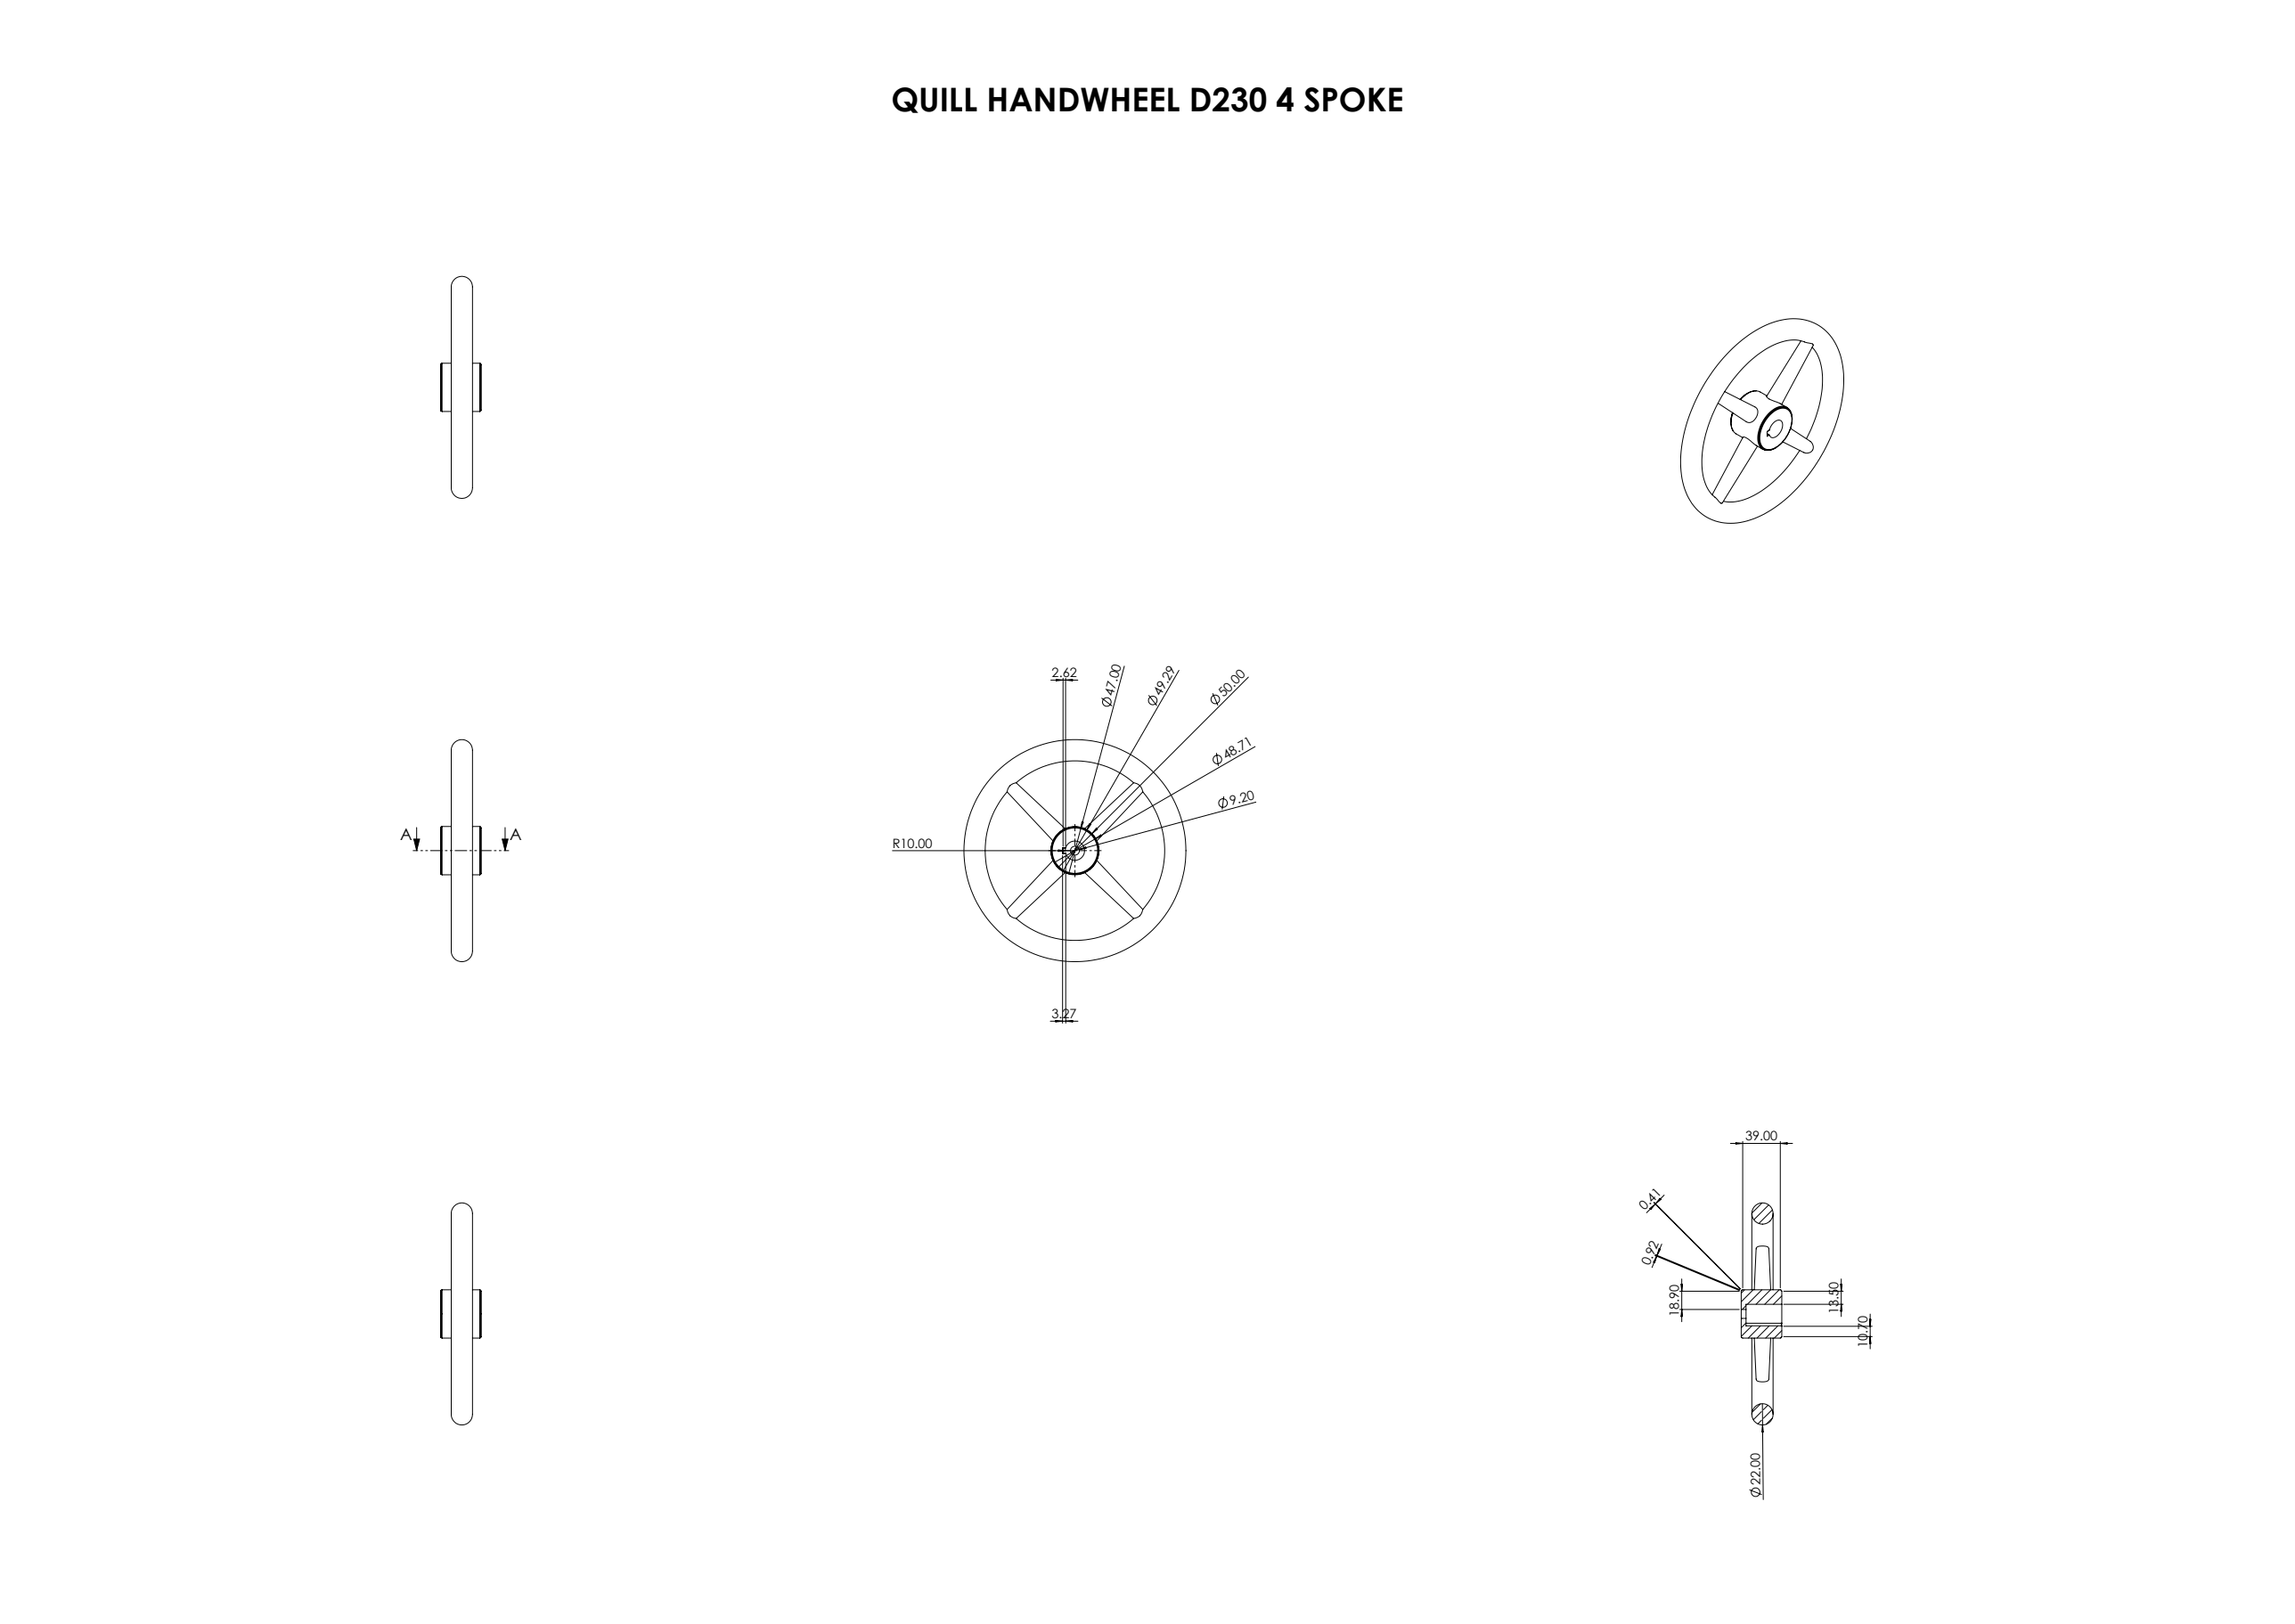
ISO-10303-21;
HEADER;
/* Generated by software containing ST-Developer
 * from STEP Tools, Inc. (www.steptools.com) 
 */

FILE_DESCRIPTION(
/* description */ (''),
/* implementation_level */ '2;1');

FILE_NAME(
/* name */ '09_Quill_Handwheel_D230_4_Spoke.step',
/* time_stamp */ '2026-10-26T03:50:32-07:00',
/* author */ (''),
/* organization */ (''),
/* preprocessor_version */ 'ST-DEVELOPER v20.2',
/* originating_system */ 'Autodesk Translation Framework v15.15.0.0',
/* authorisation */ '');

FILE_SCHEMA (('AUTOMOTIVE_DESIGN { 1 0 10303 214 3 1 1 }'));
ENDSEC;

DATA;
#10=MECHANICAL_DESIGN_GEOMETRIC_PRESENTATION_REPRESENTATION('',(#1046),#76660);
#421=B_SPLINE_CURVE_WITH_KNOTS('',3,(#49844,#49845,#49846,#49847,#49848,
#49849,#49850,#49851,#49852,#49853,#49854,#49855,#49856,#49857,#49858,#49859,
#49860,#49861),.UNSPECIFIED.,.F.,.F.,(4,2,2,2,2,2,2,2,4),(0.,0.33755490943604,
0.675109818872081,1.01195490866249,1.34879999845289,1.6856450882433,2.02249017803371,
2.36004508746975,2.69759999690579),.UNSPECIFIED.);
#422=B_SPLINE_CURVE_WITH_KNOTS('',3,(#49862,#49863,#49864,#49865,#49866,
#49867,#49868,#49869,#49870,#49871,#49872,#49873,#49874,#49875,#49876,#49877,
#49878,#49879),.UNSPECIFIED.,.F.,.F.,(4,2,2,2,2,2,2,2,4),(2.69759999690579,
3.03515490634183,3.37270981577787,3.70955490556828,4.04639999535868,4.38324508514909,
4.72009017493949,5.05764508437554,5.39519999381158),.UNSPECIFIED.);
#423=B_SPLINE_CURVE_WITH_KNOTS('',3,(#49882,#49883,#49884,#49885,#49886,
#49887,#49888,#49889,#49890,#49891,#49892,#49893,#49894,#49895,#49896,#49897,
#49898,#49899),.UNSPECIFIED.,.F.,.F.,(4,2,2,2,2,2,2,2,4),(0.,0.337554909436041,
0.675109818872083,1.01195490866249,1.34879999845289,1.6856450882433,2.0224901780337,
2.36004508746974,2.69759999690578),.UNSPECIFIED.);
#424=B_SPLINE_CURVE_WITH_KNOTS('',3,(#49900,#49901,#49902,#49903,#49904,
#49905,#49906,#49907,#49908,#49909,#49910,#49911,#49912,#49913,#49914,#49915,
#49916,#49917),.UNSPECIFIED.,.F.,.F.,(4,2,2,2,2,2,2,2,4),(2.69759999690578,
3.03515490634183,3.37270981577787,3.70955490556827,4.04639999535868,4.38324508514908,
4.72009017493949,5.05764508437553,5.39519999381157),.UNSPECIFIED.);
#425=B_SPLINE_CURVE_WITH_KNOTS('',3,(#49920,#49921,#49922,#49923,#49924,
#49925,#49926,#49927,#49928,#49929,#49930,#49931,#49932,#49933,#49934,#49935,
#49936,#49937),.UNSPECIFIED.,.F.,.F.,(4,2,2,2,2,2,2,2,4),(0.,0.337554909436041,
0.675109818872081,1.01195490866249,1.3487999984529,1.6856450882433,2.02249017803371,
2.36004508746975,2.69759999690579),.UNSPECIFIED.);
#426=B_SPLINE_CURVE_WITH_KNOTS('',3,(#49938,#49939,#49940,#49941,#49942,
#49943,#49944,#49945,#49946,#49947,#49948,#49949,#49950,#49951,#49952,#49953,
#49954,#49955),.UNSPECIFIED.,.F.,.F.,(4,2,2,2,2,2,2,2,4),(2.69759999690579,
3.03515490634183,3.37270981577787,3.70955490556828,4.04639999535869,4.3832450851491,
4.7200901749395,5.05764508437554,5.39519999381158),.UNSPECIFIED.);
#427=B_SPLINE_CURVE_WITH_KNOTS('',3,(#49958,#49959,#49960,#49961,#49962,
#49963,#49964,#49965,#49966,#49967,#49968,#49969,#49970,#49971,#49972,#49973,
#49974,#49975),.UNSPECIFIED.,.F.,.F.,(4,2,2,2,2,2,2,2,4),(0.,0.337554909436041,
0.675109818872081,1.01195490866249,1.3487999984529,1.6856450882433,2.02249017803371,
2.36004508746975,2.69759999690579),.UNSPECIFIED.);
#428=B_SPLINE_CURVE_WITH_KNOTS('',3,(#49976,#49977,#49978,#49979,#49980,
#49981,#49982,#49983,#49984,#49985,#49986,#49987,#49988,#49989,#49990,#49991,
#49992,#49993),.UNSPECIFIED.,.F.,.F.,(4,2,2,2,2,2,2,2,4),(2.69759999690579,
3.03515490634183,3.37270981577787,3.70955490556828,4.04639999535869,4.3832450851491,
4.72009017493951,5.05764508437555,5.39519999381159),.UNSPECIFIED.);
#429=B_SPLINE_CURVE_WITH_KNOTS('',3,(#50065,#50066,#50067,#50068,#50069,
#50070,#50071,#50072,#50073,#50074,#50075,#50076,#50077,#50078,#50079,#50080),
 .UNSPECIFIED.,.F.,.F.,(4,2,2,2,2,2,2,4),(-4.30443928379571,-4.2860545404295,
-4.18302089376354,-4.02031324727212,-3.73577474040229,-3.47881030687683,
-3.26117067957846,-3.22870524423984),.UNSPECIFIED.);
#430=B_SPLINE_CURVE_WITH_KNOTS('',3,(#50082,#50083,#50084,#50085,#50086,
#50087,#50088,#50089,#50090,#50091,#50092,#50093,#50094,#50095),
 .UNSPECIFIED.,.F.,.F.,(4,2,2,2,2,2,4),(-1.07597467085911,-1.02250399542755,
-0.791813858983204,-0.526066025069406,-0.242334063735881,-0.0987908890199728,
0.),.UNSPECIFIED.);
#431=B_SPLINE_CURVE_WITH_KNOTS('',3,(#50096,#50097,#50098,#50099,#50100,
#50101,#50102,#50103,#50104,#50105,#50106,#50107,#50108,#50109,#50110,#50111,
#50112,#50113,#50114,#50115,#50116,#50117,#50118,#50119),.UNSPECIFIED.,
 .F.,.F.,(4,2,2,2,2,2,2,2,2,2,2,4),(-3.22870524423984,-3.04034029687005,
-2.77983245466332,-2.48572420120637,-2.29812682077172,-2.18914179422406,
-2.09440056074871,-1.97639597697234,-1.7640763751916,-1.47308567187965,
-1.23740056701131,-1.07597467085911),.UNSPECIFIED.);
#432=B_SPLINE_CURVE_WITH_KNOTS('',3,(#50124,#50125,#50126,#50127,#50128,
#50129,#50130,#50131,#50132,#50133,#50134,#50135,#50136,#50137,#50138,#50139),
 .UNSPECIFIED.,.F.,.F.,(4,2,2,2,2,2,2,4),(-4.30443928376566,-4.28605454039955,
-4.18302089373508,-4.02031324724582,-3.73577474037948,-3.47881030685707,
-3.2611706795612,-3.22870524422297),.UNSPECIFIED.);
#433=B_SPLINE_CURVE_WITH_KNOTS('',3,(#50141,#50142,#50143,#50144,#50145,
#50146,#50147,#50148,#50149,#50150,#50151,#50152,#50153,#50154),
 .UNSPECIFIED.,.F.,.F.,(4,2,2,2,2,2,4),(-1.07597467085728,-1.02250399542586,
-0.791813858982145,-0.526066025068897,-0.242334063735757,-0.0987908890199458,
0.),.UNSPECIFIED.);
#434=B_SPLINE_CURVE_WITH_KNOTS('',3,(#50155,#50156,#50157,#50158,#50159,
#50160,#50161,#50162,#50163,#50164,#50165,#50166,#50167,#50168,#50169,#50170,
#50171,#50172,#50173,#50174,#50175,#50176,#50177,#50178),.UNSPECIFIED.,
 .F.,.F.,(4,2,2,2,2,2,2,2,2,2,2,4),(-3.22870524422297,-3.0403402968552,
-2.7798324546511,-2.48572420119689,-2.29812682076393,-2.18914179421705,
-2.09440056074233,-1.97639597696673,-1.76407637518704,-1.47308567187632,
-1.23740056700891,-1.07597467085728),.UNSPECIFIED.);
#435=B_SPLINE_CURVE_WITH_KNOTS('',3,(#50183,#50184,#50185,#50186,#50187,
#50188,#50189,#50190,#50191,#50192,#50193,#50194,#50195,#50196,#50197,#50198),
 .UNSPECIFIED.,.F.,.F.,(4,2,2,2,2,2,2,4),(-4.30443928371459,-4.28605454034862,
-4.18302089368667,-4.02031324720125,-3.73577474034113,-3.47881030682397,
-3.2611706795323,-3.22870524419465),.UNSPECIFIED.);
#436=B_SPLINE_CURVE_WITH_KNOTS('',3,(#50200,#50201,#50202,#50203,#50204,
#50205,#50206,#50207,#50208,#50209,#50210,#50211,#50212,#50213),
 .UNSPECIFIED.,.F.,.F.,(4,2,2,2,2,2,4),(-1.07597467085434,-1.02250399542317,
-0.791813858980425,-0.526066025068098,-0.242334063735552,-0.098790889019902,
0.),.UNSPECIFIED.);
#437=B_SPLINE_CURVE_WITH_KNOTS('',3,(#50214,#50215,#50216,#50217,#50218,
#50219,#50220,#50221,#50222,#50223,#50224,#50225,#50226,#50227,#50228,#50229,
#50230,#50231,#50232,#50233,#50234,#50235,#50236,#50237),.UNSPECIFIED.,
 .F.,.F.,(4,2,2,2,2,2,2,2,2,2,2,4),(-3.22870524419465,-3.04034029683025,
-2.77983245463047,-2.48572420118091,-2.2981268207507,-2.18914179420531,
-2.09440056073169,-1.97639597695723,-1.76407637517944,-1.47308567187093,
-1.23740056700507,-1.07597467085434),.UNSPECIFIED.);
#438=B_SPLINE_CURVE_WITH_KNOTS('',3,(#50242,#50243,#50244,#50245,#50246,
#50247,#50248,#50249,#50250,#50251,#50252,#50253,#50254,#50255,#50256,#50257),
 .UNSPECIFIED.,.F.,.F.,(4,2,2,2,2,2,2,4),(-4.30443928358367,-4.28605454021807,
-4.18302089356202,-4.02031324708534,-3.73577474023997,-3.47881030673541,
-3.26117067945383,-3.22870524411765),.UNSPECIFIED.);
#439=B_SPLINE_CURVE_WITH_KNOTS('',3,(#50259,#50260,#50261,#50262,#50263,
#50264,#50265,#50266,#50267,#50268,#50269,#50270,#50271,#50272),
 .UNSPECIFIED.,.F.,.F.,(4,2,2,2,2,2,4),(-1.07597467084362,-1.02250399541335,
-0.791813858973979,-0.526066025064686,-0.242334063734663,-0.0987908890197505,
0.),.UNSPECIFIED.);
#440=B_SPLINE_CURVE_WITH_KNOTS('',3,(#50273,#50274,#50275,#50276,#50277,
#50278,#50279,#50280,#50281,#50282,#50283,#50284,#50285,#50286,#50287,#50288,
#50289,#50290,#50291,#50292,#50293,#50294,#50295,#50296),.UNSPECIFIED.,
 .F.,.F.,(4,2,2,2,2,2,2,2,2,2,2,4),(-3.22870524411765,-3.04034029676145,
-2.77983245457245,-2.48572420113423,-2.29812682071072,-2.18914179416892,
-2.0944005606982,-1.976395976927,-1.76407637515459,-1.47308567185275,-1.23740056699153,
-1.07597467084362),.UNSPECIFIED.);
#1006=SHAPE_REPRESENTATION_RELATIONSHIP('SRR','None',#76743,#1026);
#1026=ADVANCED_BREP_SHAPE_REPRESENTATION('',(#1066),#76647);
#1046=STYLED_ITEM('',(#76899),#1066);
#1066=MANIFOLD_SOLID_BREP('Handwheel',#26671);
#1085=TOROIDAL_SURFACE('',#27865,10.4,1.1);
#1099=ELLIPSE('',#27852,1.41421356237309,1.);
#1100=ELLIPSE('',#27854,1.41421356237308,1.);
#1265=CYLINDRICAL_SURFACE('',#27831,2.5);
#1266=CYLINDRICAL_SURFACE('',#27859,1.);
#1267=CYLINDRICAL_SURFACE('',#27872,0.46);
#1628=FACE_BOUND('',#4742,.T.);
#1629=FACE_BOUND('',#4743,.T.);
#1630=FACE_BOUND('',#4744,.T.);
#1631=FACE_BOUND('',#4745,.T.);
#1632=FACE_BOUND('',#4751,.T.);
#1633=FACE_BOUND('',#4754,.T.);
#1634=FACE_BOUND('',#4769,.T.);
#1935=PLANE('',#27845);
#1936=PLANE('',#27849);
#1937=PLANE('',#27851);
#1938=PLANE('',#27853);
#1939=PLANE('',#27855);
#1940=PLANE('',#27856);
#1941=PLANE('',#27857);
#1942=PLANE('',#27858);
#1943=PLANE('',#27874);
#3113=FACE_OUTER_BOUND('',#4740,.T.);
#3114=FACE_OUTER_BOUND('',#4741,.T.);
#3115=FACE_OUTER_BOUND('',#4746,.T.);
#3116=FACE_OUTER_BOUND('',#4747,.T.);
#3117=FACE_OUTER_BOUND('',#4748,.T.);
#3118=FACE_OUTER_BOUND('',#4749,.T.);
#3119=FACE_OUTER_BOUND('',#4750,.T.);
#3120=FACE_OUTER_BOUND('',#4752,.T.);
#3121=FACE_OUTER_BOUND('',#4753,.T.);
#3122=FACE_OUTER_BOUND('',#4755,.T.);
#3123=FACE_OUTER_BOUND('',#4756,.T.);
#3124=FACE_OUTER_BOUND('',#4757,.T.);
#3125=FACE_OUTER_BOUND('',#4758,.T.);
#3126=FACE_OUTER_BOUND('',#4759,.T.);
#3127=FACE_OUTER_BOUND('',#4760,.T.);
#3128=FACE_OUTER_BOUND('',#4761,.T.);
#3129=FACE_OUTER_BOUND('',#4762,.T.);
#3130=FACE_OUTER_BOUND('',#4763,.T.);
#3131=FACE_OUTER_BOUND('',#4764,.T.);
#3132=FACE_OUTER_BOUND('',#4765,.T.);
#3133=FACE_OUTER_BOUND('',#4766,.T.);
#3134=FACE_OUTER_BOUND('',#4767,.T.);
#3135=FACE_OUTER_BOUND('',#4768,.T.);
#4740=EDGE_LOOP('',(#20043,#20044,#20045,#20046,#20047,#20048));
#4741=EDGE_LOOP('',(#20049,#20050,#20051,#20052,#20053,#20054));
#4742=EDGE_LOOP('',(#20055,#20056));
#4743=EDGE_LOOP('',(#20057,#20058));
#4744=EDGE_LOOP('',(#20059,#20060));
#4745=EDGE_LOOP('',(#20061,#20062));
#4746=EDGE_LOOP('',(#20063,#20064,#20065,#20066,#20067,#20068));
#4747=EDGE_LOOP('',(#20069,#20070,#20071,#20072,#20073,#20074));
#4748=EDGE_LOOP('',(#20075,#20076,#20077,#20078,#20079,#20080));
#4749=EDGE_LOOP('',(#20081,#20082,#20083,#20084,#20085));
#4750=EDGE_LOOP('',(#20086));
#4751=EDGE_LOOP('',(#20087));
#4752=EDGE_LOOP('',(#20088,#20089,#20090,#20091,#20092));
#4753=EDGE_LOOP('',(#20093));
#4754=EDGE_LOOP('',(#20094,#20095,#20096,#20097));
#4755=EDGE_LOOP('',(#20098,#20099,#20100,#20101));
#4756=EDGE_LOOP('',(#20102,#20103,#20104,#20105));
#4757=EDGE_LOOP('',(#20106,#20107,#20108,#20109));
#4758=EDGE_LOOP('',(#20110,#20111,#20112,#20113));
#4759=EDGE_LOOP('',(#20114,#20115,#20116,#20117));
#4760=EDGE_LOOP('',(#20118,#20119,#20120,#20121));
#4761=EDGE_LOOP('',(#20122,#20123,#20124,#20125,#20126,#20127));
#4762=EDGE_LOOP('',(#20128,#20129,#20130,#20131,#20132,#20133,#20134));
#4763=EDGE_LOOP('',(#20135,#20136,#20137,#20138,#20139,#20140,#20141));
#4764=EDGE_LOOP('',(#20142,#20143,#20144,#20145,#20146,#20147,#20148));
#4765=EDGE_LOOP('',(#20149,#20150,#20151,#20152,#20153,#20154,#20155));
#4766=EDGE_LOOP('',(#20156,#20157,#20158,#20159,#20160,#20161,#20162,#20163,
#20164,#20165,#20166,#20167,#20168,#20169,#20170,#20171,#20172,#20173,#20174,
#20175,#20176,#20177,#20178,#20179));
#4767=EDGE_LOOP('',(#20180,#20181,#20182,#20183));
#4768=EDGE_LOOP('',(#20184,#20185,#20186,#20187));
#4769=EDGE_LOOP('',(#20188));
#6066=CIRCLE('',#27827,2.46464466094067);
#6067=CIRCLE('',#27828,2.46464466094067);
#6068=CIRCLE('',#27829,2.5);
#6069=CIRCLE('',#27830,2.5);
#6070=CIRCLE('',#27832,2.5);
#6071=CIRCLE('',#27833,2.5);
#6072=CIRCLE('',#27835,2.43535533905933);
#6073=CIRCLE('',#27836,2.43535533905933);
#6074=CIRCLE('',#27838,2.46464466094067);
#6075=CIRCLE('',#27839,2.46464466094067);
#6076=CIRCLE('',#27841,2.43535533905933);
#6077=CIRCLE('',#27842,2.43535533905933);
#6078=CIRCLE('',#27844,2.35);
#6079=CIRCLE('',#27846,0.46);
#6080=CIRCLE('',#27848,2.35);
#6081=CIRCLE('',#27850,1.);
#6082=CIRCLE('',#27860,1.);
#6083=CIRCLE('',#27866,1.1);
#6084=CIRCLE('',#27867,9.3);
#6085=CIRCLE('',#27868,9.3);
#6086=CIRCLE('',#27869,9.3);
#6087=CIRCLE('',#27870,9.3);
#6088=CIRCLE('',#27871,9.3);
#6089=CIRCLE('',#27873,0.46);
#7429=LINE('',#49832,#9585);
#7430=LINE('',#49838,#9586);
#7431=LINE('',#49999,#9587);
#7432=LINE('',#50002,#9588);
#7433=LINE('',#50008,#9589);
#7434=LINE('',#50014,#9590);
#7435=LINE('',#50022,#9591);
#7436=LINE('',#50026,#9592);
#7437=LINE('',#50030,#9593);
#7438=LINE('',#50031,#9594);
#7439=LINE('',#50035,#9595);
#7440=LINE('',#50037,#9596);
#7441=LINE('',#50042,#9597);
#7442=LINE('',#50043,#9598);
#7443=LINE('',#50045,#9599);
#7444=LINE('',#50048,#9600);
#7445=LINE('',#50050,#9601);
#7446=LINE('',#50051,#9602);
#7447=LINE('',#50054,#9603);
#7448=LINE('',#50055,#9604);
#7449=LINE('',#50058,#9605);
#7450=LINE('',#50059,#9606);
#7451=LINE('',#50120,#9607);
#7452=LINE('',#50179,#9608);
#7453=LINE('',#50238,#9609);
#7454=LINE('',#50297,#9610);
#7455=LINE('',#50309,#9611);
#9585=VECTOR('',#32030,2.48232233047034);
#9586=VECTOR('',#32037,2.5);
#9587=VECTOR('',#32048,2.45);
#9588=VECTOR('',#32051,2.48232233047034);
#9589=VECTOR('',#32058,2.45);
#9590=VECTOR('',#32065,2.39267766952966);
#9591=VECTOR('',#32076,2.39267766952966);
#9592=VECTOR('',#32079,1.);
#9593=VECTOR('',#32082,1.);
#9594=VECTOR('',#32083,1.);
#9595=VECTOR('',#32086,1.);
#9596=VECTOR('',#32089,1.);
#9597=VECTOR('',#32094,1.);
#9598=VECTOR('',#32095,1.);
#9599=VECTOR('',#32098,1.);
#9600=VECTOR('',#32101,1.);
#9601=VECTOR('',#32102,1.);
#9602=VECTOR('',#32103,1.);
#9603=VECTOR('',#32106,1.);
#9604=VECTOR('',#32107,1.);
#9605=VECTOR('',#32110,1.);
#9606=VECTOR('',#32111,1.);
#9607=VECTOR('',#32118,0.775);
#9608=VECTOR('',#32121,0.775);
#9609=VECTOR('',#32124,0.775000000000002);
#9610=VECTOR('',#32127,0.774999999999997);
#9611=VECTOR('',#32146,0.46);
#11797=VERTEX_POINT('',#49827);
#11798=VERTEX_POINT('',#49828);
#11799=VERTEX_POINT('',#49831);
#11800=VERTEX_POINT('',#49833);
#11801=VERTEX_POINT('',#49837);
#11802=VERTEX_POINT('',#49839);
#11803=VERTEX_POINT('',#49842);
#11804=VERTEX_POINT('',#49843);
#11805=VERTEX_POINT('',#49880);
#11806=VERTEX_POINT('',#49881);
#11807=VERTEX_POINT('',#49918);
#11808=VERTEX_POINT('',#49919);
#11809=VERTEX_POINT('',#49956);
#11810=VERTEX_POINT('',#49957);
#11811=VERTEX_POINT('',#49995);
#11812=VERTEX_POINT('',#49996);
#11813=VERTEX_POINT('',#50001);
#11814=VERTEX_POINT('',#50003);
#11815=VERTEX_POINT('',#50007);
#11816=VERTEX_POINT('',#50009);
#11817=VERTEX_POINT('',#50013);
#11818=VERTEX_POINT('',#50017);
#11819=VERTEX_POINT('',#50020);
#11820=VERTEX_POINT('',#50024);
#11821=VERTEX_POINT('',#50025);
#11822=VERTEX_POINT('',#50027);
#11823=VERTEX_POINT('',#50029);
#11824=VERTEX_POINT('',#50033);
#11825=VERTEX_POINT('',#50034);
#11826=VERTEX_POINT('',#50039);
#11827=VERTEX_POINT('',#50041);
#11828=VERTEX_POINT('',#50047);
#11829=VERTEX_POINT('',#50049);
#11830=VERTEX_POINT('',#50053);
#11831=VERTEX_POINT('',#50057);
#11832=VERTEX_POINT('',#50063);
#11833=VERTEX_POINT('',#50064);
#11834=VERTEX_POINT('',#50081);
#11835=VERTEX_POINT('',#50122);
#11836=VERTEX_POINT('',#50123);
#11837=VERTEX_POINT('',#50140);
#11838=VERTEX_POINT('',#50181);
#11839=VERTEX_POINT('',#50182);
#11840=VERTEX_POINT('',#50199);
#11841=VERTEX_POINT('',#50240);
#11842=VERTEX_POINT('',#50241);
#11843=VERTEX_POINT('',#50258);
#11844=VERTEX_POINT('',#50299);
#11845=VERTEX_POINT('',#50307);
#14744=EDGE_CURVE('',#11797,#11798,#6066,.T.);
#14745=EDGE_CURVE('',#11798,#11797,#6067,.T.);
#14746=EDGE_CURVE('',#11797,#11799,#7429,.T.);
#14747=EDGE_CURVE('',#11799,#11800,#6068,.T.);
#14748=EDGE_CURVE('',#11800,#11799,#6069,.T.);
#14749=EDGE_CURVE('',#11800,#11801,#7430,.T.);
#14750=EDGE_CURVE('',#11802,#11801,#6070,.T.);
#14751=EDGE_CURVE('',#11801,#11802,#6071,.T.);
#14752=EDGE_CURVE('',#11803,#11804,#421,.T.);
#14753=EDGE_CURVE('',#11804,#11803,#422,.T.);
#14754=EDGE_CURVE('',#11805,#11806,#423,.T.);
#14755=EDGE_CURVE('',#11806,#11805,#424,.T.);
#14756=EDGE_CURVE('',#11807,#11808,#425,.T.);
#14757=EDGE_CURVE('',#11808,#11807,#426,.T.);
#14758=EDGE_CURVE('',#11809,#11810,#427,.T.);
#14759=EDGE_CURVE('',#11810,#11809,#428,.T.);
#14760=EDGE_CURVE('',#11811,#11812,#6072,.T.);
#14761=EDGE_CURVE('',#11812,#11811,#6073,.T.);
#14762=EDGE_CURVE('',#11812,#11798,#7431,.T.);
#14763=EDGE_CURVE('',#11802,#11813,#7432,.T.);
#14764=EDGE_CURVE('',#11813,#11814,#6074,.T.);
#14765=EDGE_CURVE('',#11814,#11813,#6075,.T.);
#14766=EDGE_CURVE('',#11814,#11815,#7433,.T.);
#14767=EDGE_CURVE('',#11816,#11815,#6076,.T.);
#14768=EDGE_CURVE('',#11815,#11816,#6077,.T.);
#14769=EDGE_CURVE('',#11816,#11817,#7434,.T.);
#14770=EDGE_CURVE('',#11817,#11817,#6078,.T.);
#14771=EDGE_CURVE('',#11818,#11818,#6079,.T.);
#14772=EDGE_CURVE('',#11819,#11819,#6080,.T.);
#14773=EDGE_CURVE('',#11819,#11811,#7435,.T.);
#14774=EDGE_CURVE('',#11820,#11821,#7436,.T.);
#14775=EDGE_CURVE('',#11822,#11820,#6081,.T.);
#14776=EDGE_CURVE('',#11823,#11822,#7437,.T.);
#14777=EDGE_CURVE('',#11821,#11823,#7438,.T.);
#14778=EDGE_CURVE('',#11824,#11825,#7439,.T.);
#14779=EDGE_CURVE('',#11825,#11820,#1099,.T.);
#14780=EDGE_CURVE('',#11821,#11824,#7440,.T.);
#14781=EDGE_CURVE('',#11822,#11826,#1100,.T.);
#14782=EDGE_CURVE('',#11826,#11827,#7441,.T.);
#14783=EDGE_CURVE('',#11827,#11823,#7442,.T.);
#14784=EDGE_CURVE('',#11827,#11824,#7443,.T.);
#14785=EDGE_CURVE('',#11828,#11827,#7444,.T.);
#14786=EDGE_CURVE('',#11829,#11828,#7445,.T.);
#14787=EDGE_CURVE('',#11824,#11829,#7446,.T.);
#14788=EDGE_CURVE('',#11830,#11826,#7447,.T.);
#14789=EDGE_CURVE('',#11828,#11830,#7448,.T.);
#14790=EDGE_CURVE('',#11829,#11831,#7449,.T.);
#14791=EDGE_CURVE('',#11825,#11831,#7450,.T.);
#14792=EDGE_CURVE('',#11830,#11831,#6082,.T.);
#14793=EDGE_CURVE('',#11832,#11833,#429,.T.);
#14794=EDGE_CURVE('',#11834,#11832,#430,.T.);
#14795=EDGE_CURVE('',#11833,#11834,#431,.T.);
#14796=EDGE_CURVE('',#11833,#11804,#7451,.T.);
#14797=EDGE_CURVE('',#11835,#11836,#432,.T.);
#14798=EDGE_CURVE('',#11837,#11835,#433,.T.);
#14799=EDGE_CURVE('',#11836,#11837,#434,.T.);
#14800=EDGE_CURVE('',#11836,#11806,#7452,.T.);
#14801=EDGE_CURVE('',#11838,#11839,#435,.T.);
#14802=EDGE_CURVE('',#11840,#11838,#436,.T.);
#14803=EDGE_CURVE('',#11839,#11840,#437,.T.);
#14804=EDGE_CURVE('',#11839,#11808,#7453,.T.);
#14805=EDGE_CURVE('',#11841,#11842,#438,.T.);
#14806=EDGE_CURVE('',#11843,#11841,#439,.T.);
#14807=EDGE_CURVE('',#11842,#11843,#440,.T.);
#14808=EDGE_CURVE('',#11842,#11810,#7454,.T.);
#14809=EDGE_CURVE('',#11844,#11844,#6083,.T.);
#14810=EDGE_CURVE('',#11839,#11844,#6084,.T.);
#14811=EDGE_CURVE('',#11836,#11840,#6085,.T.);
#14812=EDGE_CURVE('',#11833,#11837,#6086,.T.);
#14813=EDGE_CURVE('',#11842,#11834,#6087,.T.);
#14814=EDGE_CURVE('',#11844,#11843,#6088,.T.);
#14815=EDGE_CURVE('',#11845,#11845,#6089,.T.);
#14816=EDGE_CURVE('',#11845,#11818,#7455,.T.);
#20043=ORIENTED_EDGE('',*,*,#14744,.T.);
#20044=ORIENTED_EDGE('',*,*,#14745,.T.);
#20045=ORIENTED_EDGE('',*,*,#14746,.T.);
#20046=ORIENTED_EDGE('',*,*,#14747,.T.);
#20047=ORIENTED_EDGE('',*,*,#14748,.T.);
#20048=ORIENTED_EDGE('',*,*,#14746,.F.);
#20049=ORIENTED_EDGE('',*,*,#14747,.F.);
#20050=ORIENTED_EDGE('',*,*,#14748,.F.);
#20051=ORIENTED_EDGE('',*,*,#14749,.T.);
#20052=ORIENTED_EDGE('',*,*,#14750,.F.);
#20053=ORIENTED_EDGE('',*,*,#14751,.F.);
#20054=ORIENTED_EDGE('',*,*,#14749,.F.);
#20055=ORIENTED_EDGE('',*,*,#14752,.T.);
#20056=ORIENTED_EDGE('',*,*,#14753,.T.);
#20057=ORIENTED_EDGE('',*,*,#14754,.T.);
#20058=ORIENTED_EDGE('',*,*,#14755,.T.);
#20059=ORIENTED_EDGE('',*,*,#14756,.T.);
#20060=ORIENTED_EDGE('',*,*,#14757,.T.);
#20061=ORIENTED_EDGE('',*,*,#14758,.T.);
#20062=ORIENTED_EDGE('',*,*,#14759,.T.);
#20063=ORIENTED_EDGE('',*,*,#14760,.F.);
#20064=ORIENTED_EDGE('',*,*,#14761,.F.);
#20065=ORIENTED_EDGE('',*,*,#14762,.T.);
#20066=ORIENTED_EDGE('',*,*,#14744,.F.);
#20067=ORIENTED_EDGE('',*,*,#14745,.F.);
#20068=ORIENTED_EDGE('',*,*,#14762,.F.);
#20069=ORIENTED_EDGE('',*,*,#14750,.T.);
#20070=ORIENTED_EDGE('',*,*,#14751,.T.);
#20071=ORIENTED_EDGE('',*,*,#14763,.T.);
#20072=ORIENTED_EDGE('',*,*,#14764,.T.);
#20073=ORIENTED_EDGE('',*,*,#14765,.T.);
#20074=ORIENTED_EDGE('',*,*,#14763,.F.);
#20075=ORIENTED_EDGE('',*,*,#14764,.F.);
#20076=ORIENTED_EDGE('',*,*,#14765,.F.);
#20077=ORIENTED_EDGE('',*,*,#14766,.T.);
#20078=ORIENTED_EDGE('',*,*,#14767,.F.);
#20079=ORIENTED_EDGE('',*,*,#14768,.F.);
#20080=ORIENTED_EDGE('',*,*,#14766,.F.);
#20081=ORIENTED_EDGE('',*,*,#14767,.T.);
#20082=ORIENTED_EDGE('',*,*,#14768,.T.);
#20083=ORIENTED_EDGE('',*,*,#14769,.T.);
#20084=ORIENTED_EDGE('',*,*,#14770,.T.);
#20085=ORIENTED_EDGE('',*,*,#14769,.F.);
#20086=ORIENTED_EDGE('',*,*,#14770,.F.);
#20087=ORIENTED_EDGE('',*,*,#14771,.T.);
#20088=ORIENTED_EDGE('',*,*,#14772,.T.);
#20089=ORIENTED_EDGE('',*,*,#14773,.T.);
#20090=ORIENTED_EDGE('',*,*,#14760,.T.);
#20091=ORIENTED_EDGE('',*,*,#14761,.T.);
#20092=ORIENTED_EDGE('',*,*,#14773,.F.);
#20093=ORIENTED_EDGE('',*,*,#14772,.F.);
#20094=ORIENTED_EDGE('',*,*,#14774,.F.);
#20095=ORIENTED_EDGE('',*,*,#14775,.F.);
#20096=ORIENTED_EDGE('',*,*,#14776,.F.);
#20097=ORIENTED_EDGE('',*,*,#14777,.F.);
#20098=ORIENTED_EDGE('',*,*,#14778,.T.);
#20099=ORIENTED_EDGE('',*,*,#14779,.T.);
#20100=ORIENTED_EDGE('',*,*,#14774,.T.);
#20101=ORIENTED_EDGE('',*,*,#14780,.T.);
#20102=ORIENTED_EDGE('',*,*,#14776,.T.);
#20103=ORIENTED_EDGE('',*,*,#14781,.T.);
#20104=ORIENTED_EDGE('',*,*,#14782,.T.);
#20105=ORIENTED_EDGE('',*,*,#14783,.T.);
#20106=ORIENTED_EDGE('',*,*,#14777,.T.);
#20107=ORIENTED_EDGE('',*,*,#14783,.F.);
#20108=ORIENTED_EDGE('',*,*,#14784,.T.);
#20109=ORIENTED_EDGE('',*,*,#14780,.F.);
#20110=ORIENTED_EDGE('',*,*,#14784,.F.);
#20111=ORIENTED_EDGE('',*,*,#14785,.F.);
#20112=ORIENTED_EDGE('',*,*,#14786,.F.);
#20113=ORIENTED_EDGE('',*,*,#14787,.F.);
#20114=ORIENTED_EDGE('',*,*,#14782,.F.);
#20115=ORIENTED_EDGE('',*,*,#14788,.F.);
#20116=ORIENTED_EDGE('',*,*,#14789,.F.);
#20117=ORIENTED_EDGE('',*,*,#14785,.T.);
#20118=ORIENTED_EDGE('',*,*,#14778,.F.);
#20119=ORIENTED_EDGE('',*,*,#14787,.T.);
#20120=ORIENTED_EDGE('',*,*,#14790,.T.);
#20121=ORIENTED_EDGE('',*,*,#14791,.F.);
#20122=ORIENTED_EDGE('',*,*,#14779,.F.);
#20123=ORIENTED_EDGE('',*,*,#14791,.T.);
#20124=ORIENTED_EDGE('',*,*,#14792,.F.);
#20125=ORIENTED_EDGE('',*,*,#14788,.T.);
#20126=ORIENTED_EDGE('',*,*,#14781,.F.);
#20127=ORIENTED_EDGE('',*,*,#14775,.T.);
#20128=ORIENTED_EDGE('',*,*,#14793,.F.);
#20129=ORIENTED_EDGE('',*,*,#14794,.F.);
#20130=ORIENTED_EDGE('',*,*,#14795,.F.);
#20131=ORIENTED_EDGE('',*,*,#14796,.T.);
#20132=ORIENTED_EDGE('',*,*,#14752,.F.);
#20133=ORIENTED_EDGE('',*,*,#14753,.F.);
#20134=ORIENTED_EDGE('',*,*,#14796,.F.);
#20135=ORIENTED_EDGE('',*,*,#14797,.F.);
#20136=ORIENTED_EDGE('',*,*,#14798,.F.);
#20137=ORIENTED_EDGE('',*,*,#14799,.F.);
#20138=ORIENTED_EDGE('',*,*,#14800,.T.);
#20139=ORIENTED_EDGE('',*,*,#14754,.F.);
#20140=ORIENTED_EDGE('',*,*,#14755,.F.);
#20141=ORIENTED_EDGE('',*,*,#14800,.F.);
#20142=ORIENTED_EDGE('',*,*,#14801,.F.);
#20143=ORIENTED_EDGE('',*,*,#14802,.F.);
#20144=ORIENTED_EDGE('',*,*,#14803,.F.);
#20145=ORIENTED_EDGE('',*,*,#14804,.T.);
#20146=ORIENTED_EDGE('',*,*,#14756,.F.);
#20147=ORIENTED_EDGE('',*,*,#14757,.F.);
#20148=ORIENTED_EDGE('',*,*,#14804,.F.);
#20149=ORIENTED_EDGE('',*,*,#14805,.F.);
#20150=ORIENTED_EDGE('',*,*,#14806,.F.);
#20151=ORIENTED_EDGE('',*,*,#14807,.F.);
#20152=ORIENTED_EDGE('',*,*,#14808,.T.);
#20153=ORIENTED_EDGE('',*,*,#14758,.F.);
#20154=ORIENTED_EDGE('',*,*,#14759,.F.);
#20155=ORIENTED_EDGE('',*,*,#14808,.F.);
#20156=ORIENTED_EDGE('',*,*,#14809,.T.);
#20157=ORIENTED_EDGE('',*,*,#14810,.F.);
#20158=ORIENTED_EDGE('',*,*,#14803,.T.);
#20159=ORIENTED_EDGE('',*,*,#14811,.F.);
#20160=ORIENTED_EDGE('',*,*,#14799,.T.);
#20161=ORIENTED_EDGE('',*,*,#14812,.F.);
#20162=ORIENTED_EDGE('',*,*,#14795,.T.);
#20163=ORIENTED_EDGE('',*,*,#14813,.F.);
#20164=ORIENTED_EDGE('',*,*,#14807,.T.);
#20165=ORIENTED_EDGE('',*,*,#14814,.F.);
#20166=ORIENTED_EDGE('',*,*,#14809,.F.);
#20167=ORIENTED_EDGE('',*,*,#14814,.T.);
#20168=ORIENTED_EDGE('',*,*,#14806,.T.);
#20169=ORIENTED_EDGE('',*,*,#14805,.T.);
#20170=ORIENTED_EDGE('',*,*,#14813,.T.);
#20171=ORIENTED_EDGE('',*,*,#14794,.T.);
#20172=ORIENTED_EDGE('',*,*,#14793,.T.);
#20173=ORIENTED_EDGE('',*,*,#14812,.T.);
#20174=ORIENTED_EDGE('',*,*,#14798,.T.);
#20175=ORIENTED_EDGE('',*,*,#14797,.T.);
#20176=ORIENTED_EDGE('',*,*,#14811,.T.);
#20177=ORIENTED_EDGE('',*,*,#14802,.T.);
#20178=ORIENTED_EDGE('',*,*,#14801,.T.);
#20179=ORIENTED_EDGE('',*,*,#14810,.T.);
#20180=ORIENTED_EDGE('',*,*,#14815,.T.);
#20181=ORIENTED_EDGE('',*,*,#14816,.T.);
#20182=ORIENTED_EDGE('',*,*,#14771,.F.);
#20183=ORIENTED_EDGE('',*,*,#14816,.F.);
#20184=ORIENTED_EDGE('',*,*,#14792,.T.);
#20185=ORIENTED_EDGE('',*,*,#14790,.F.);
#20186=ORIENTED_EDGE('',*,*,#14786,.T.);
#20187=ORIENTED_EDGE('',*,*,#14789,.T.);
#20188=ORIENTED_EDGE('',*,*,#14815,.F.);
#25045=CONICAL_SURFACE('',#27826,2.48232233047034,0.392699081698724);
#25046=CONICAL_SURFACE('',#27834,2.45,0.785398163397451);
#25047=CONICAL_SURFACE('',#27837,2.48232233047034,0.392699081698723);
#25048=CONICAL_SURFACE('',#27840,2.45,0.785398163397449);
#25049=CONICAL_SURFACE('',#27843,2.39267766952966,1.17809724509617);
#25050=CONICAL_SURFACE('',#27847,2.39267766952966,1.17809724509617);
#25051=CONICAL_SURFACE('',#27861,0.775,0.0320403135474668);
#25052=CONICAL_SURFACE('',#27862,0.775,0.0320403135474668);
#25053=CONICAL_SURFACE('',#27863,0.775000000000002,0.0320403135474665);
#25054=CONICAL_SURFACE('',#27864,0.774999999999997,0.032040313547468);
#25701=ADVANCED_FACE('',(#3113),#25045,.T.);
#25702=ADVANCED_FACE('',(#3114,#1628,#1629,#1630,#1631),#1265,.T.);
#25703=ADVANCED_FACE('',(#3115),#25046,.T.);
#25704=ADVANCED_FACE('',(#3116),#25047,.T.);
#25705=ADVANCED_FACE('',(#3117),#25048,.T.);
#25706=ADVANCED_FACE('',(#3118),#25049,.T.);
#25707=ADVANCED_FACE('',(#3119,#1632),#1935,.T.);
#25708=ADVANCED_FACE('',(#3120),#25050,.T.);
#25709=ADVANCED_FACE('',(#3121,#1633),#1936,.T.);
#25710=ADVANCED_FACE('',(#3122),#1937,.T.);
#25711=ADVANCED_FACE('',(#3123),#1938,.T.);
#25712=ADVANCED_FACE('',(#3124),#1939,.T.);
#25713=ADVANCED_FACE('',(#3125),#1940,.F.);
#25714=ADVANCED_FACE('',(#3126),#1941,.F.);
#25715=ADVANCED_FACE('',(#3127),#1942,.F.);
#25716=ADVANCED_FACE('',(#3128),#1266,.F.);
#25717=ADVANCED_FACE('',(#3129),#25051,.T.);
#25718=ADVANCED_FACE('',(#3130),#25052,.T.);
#25719=ADVANCED_FACE('',(#3131),#25053,.T.);
#25720=ADVANCED_FACE('',(#3132),#25054,.T.);
#25721=ADVANCED_FACE('',(#3133),#1085,.T.);
#25722=ADVANCED_FACE('',(#3134),#1267,.F.);
#25723=ADVANCED_FACE('',(#3135,#1634),#1943,.T.);
#26671=CLOSED_SHELL('',(#25701,#25702,#25703,#25704,#25705,#25706,#25707,
#25708,#25709,#25710,#25711,#25712,#25713,#25714,#25715,#25716,#25717,#25718,
#25719,#25720,#25721,#25722,#25723));
#27825=AXIS2_PLACEMENT_3D('',#49825,#32022,#32023);
#27826=AXIS2_PLACEMENT_3D('',#49826,#32024,#32025);
#27827=AXIS2_PLACEMENT_3D('',#49829,#32026,#32027);
#27828=AXIS2_PLACEMENT_3D('',#49830,#32028,#32029);
#27829=AXIS2_PLACEMENT_3D('',#49834,#32031,#32032);
#27830=AXIS2_PLACEMENT_3D('',#49835,#32033,#32034);
#27831=AXIS2_PLACEMENT_3D('',#49836,#32035,#32036);
#27832=AXIS2_PLACEMENT_3D('',#49840,#32038,#32039);
#27833=AXIS2_PLACEMENT_3D('',#49841,#32040,#32041);
#27834=AXIS2_PLACEMENT_3D('',#49994,#32042,#32043);
#27835=AXIS2_PLACEMENT_3D('',#49997,#32044,#32045);
#27836=AXIS2_PLACEMENT_3D('',#49998,#32046,#32047);
#27837=AXIS2_PLACEMENT_3D('',#50000,#32049,#32050);
#27838=AXIS2_PLACEMENT_3D('',#50004,#32052,#32053);
#27839=AXIS2_PLACEMENT_3D('',#50005,#32054,#32055);
#27840=AXIS2_PLACEMENT_3D('',#50006,#32056,#32057);
#27841=AXIS2_PLACEMENT_3D('',#50010,#32059,#32060);
#27842=AXIS2_PLACEMENT_3D('',#50011,#32061,#32062);
#27843=AXIS2_PLACEMENT_3D('',#50012,#32063,#32064);
#27844=AXIS2_PLACEMENT_3D('',#50015,#32066,#32067);
#27845=AXIS2_PLACEMENT_3D('',#50016,#32068,#32069);
#27846=AXIS2_PLACEMENT_3D('',#50018,#32070,#32071);
#27847=AXIS2_PLACEMENT_3D('',#50019,#32072,#32073);
#27848=AXIS2_PLACEMENT_3D('',#50021,#32074,#32075);
#27849=AXIS2_PLACEMENT_3D('',#50023,#32077,#32078);
#27850=AXIS2_PLACEMENT_3D('',#50028,#32080,#32081);
#27851=AXIS2_PLACEMENT_3D('',#50032,#32084,#32085);
#27852=AXIS2_PLACEMENT_3D('',#50036,#32087,#32088);
#27853=AXIS2_PLACEMENT_3D('',#50038,#32090,#32091);
#27854=AXIS2_PLACEMENT_3D('',#50040,#32092,#32093);
#27855=AXIS2_PLACEMENT_3D('',#50044,#32096,#32097);
#27856=AXIS2_PLACEMENT_3D('',#50046,#32099,#32100);
#27857=AXIS2_PLACEMENT_3D('',#50052,#32104,#32105);
#27858=AXIS2_PLACEMENT_3D('',#50056,#32108,#32109);
#27859=AXIS2_PLACEMENT_3D('',#50060,#32112,#32113);
#27860=AXIS2_PLACEMENT_3D('',#50061,#32114,#32115);
#27861=AXIS2_PLACEMENT_3D('',#50062,#32116,#32117);
#27862=AXIS2_PLACEMENT_3D('',#50121,#32119,#32120);
#27863=AXIS2_PLACEMENT_3D('',#50180,#32122,#32123);
#27864=AXIS2_PLACEMENT_3D('',#50239,#32125,#32126);
#27865=AXIS2_PLACEMENT_3D('',#50298,#32128,#32129);
#27866=AXIS2_PLACEMENT_3D('',#50300,#32130,#32131);
#27867=AXIS2_PLACEMENT_3D('',#50301,#32132,#32133);
#27868=AXIS2_PLACEMENT_3D('',#50302,#32134,#32135);
#27869=AXIS2_PLACEMENT_3D('',#50303,#32136,#32137);
#27870=AXIS2_PLACEMENT_3D('',#50304,#32138,#32139);
#27871=AXIS2_PLACEMENT_3D('',#50305,#32140,#32141);
#27872=AXIS2_PLACEMENT_3D('',#50306,#32142,#32143);
#27873=AXIS2_PLACEMENT_3D('',#50308,#32144,#32145);
#27874=AXIS2_PLACEMENT_3D('',#50310,#32147,#32148);
#32022=DIRECTION('axis',(0.,0.,1.));
#32023=DIRECTION('refdir',(1.,0.,0.));
#32024=DIRECTION('center_axis',(-1.,0.,0.));
#32025=DIRECTION('ref_axis',(0.,-1.,0.));
#32026=DIRECTION('center_axis',(-1.,0.,0.));
#32027=DIRECTION('ref_axis',(0.,-1.,0.));
#32028=DIRECTION('center_axis',(-1.,0.,0.));
#32029=DIRECTION('ref_axis',(0.,-1.,0.));
#32030=DIRECTION('',(-0.923879532511287,0.38268343236509,4.6865204053263E-17));
#32031=DIRECTION('center_axis',(1.,0.,0.));
#32032=DIRECTION('ref_axis',(0.,-1.,0.));
#32033=DIRECTION('center_axis',(1.,0.,0.));
#32034=DIRECTION('ref_axis',(0.,-1.,0.));
#32035=DIRECTION('center_axis',(1.,0.,0.));
#32036=DIRECTION('ref_axis',(0.,1.,0.));
#32037=DIRECTION('',(-1.,0.,0.));
#32038=DIRECTION('center_axis',(-1.,0.,0.));
#32039=DIRECTION('ref_axis',(0.,-1.,0.));
#32040=DIRECTION('center_axis',(-1.,0.,0.));
#32041=DIRECTION('ref_axis',(0.,-1.,0.));
#32042=DIRECTION('center_axis',(-1.,0.,0.));
#32043=DIRECTION('ref_axis',(0.,1.,0.));
#32044=DIRECTION('center_axis',(1.,0.,-3.64701776966638E-16));
#32045=DIRECTION('ref_axis',(0.,-1.,0.));
#32046=DIRECTION('center_axis',(1.,0.,-3.64701776966638E-16));
#32047=DIRECTION('ref_axis',(0.,-1.,0.));
#32048=DIRECTION('',(-0.707106781186546,-0.707106781186549,-8.65956056235495E-17));
#32049=DIRECTION('center_axis',(1.,0.,0.));
#32050=DIRECTION('ref_axis',(0.,-1.,0.));
#32051=DIRECTION('',(-0.923879532511287,-0.382683432365088,-4.68652040532628E-17));
#32052=DIRECTION('center_axis',(1.,0.,1.35137901485737E-16));
#32053=DIRECTION('ref_axis',(0.,-1.,0.));
#32054=DIRECTION('center_axis',(1.,0.,1.35137901485737E-16));
#32055=DIRECTION('ref_axis',(0.,-1.,0.));
#32056=DIRECTION('center_axis',(1.,0.,0.));
#32057=DIRECTION('ref_axis',(0.,1.,0.));
#32058=DIRECTION('',(-0.707106781186547,0.707106781186548,8.65956056235494E-17));
#32059=DIRECTION('center_axis',(-1.,0.,-4.55877221208297E-16));
#32060=DIRECTION('ref_axis',(0.,-1.,0.));
#32061=DIRECTION('center_axis',(-1.,0.,-4.55877221208297E-16));
#32062=DIRECTION('ref_axis',(0.,-1.,0.));
#32063=DIRECTION('center_axis',(1.,0.,0.));
#32064=DIRECTION('ref_axis',(0.,-1.,0.));
#32065=DIRECTION('',(-0.382683432365089,-0.923879532511287,-1.1314261122877E-16));
#32066=DIRECTION('center_axis',(1.,0.,0.));
#32067=DIRECTION('ref_axis',(0.,-1.,0.));
#32068=DIRECTION('center_axis',(-1.,0.,0.));
#32069=DIRECTION('ref_axis',(0.,0.,1.));
#32070=DIRECTION('center_axis',(1.,0.,0.));
#32071=DIRECTION('ref_axis',(0.,0.,-1.));
#32072=DIRECTION('center_axis',(-1.,0.,0.));
#32073=DIRECTION('ref_axis',(0.,-1.,0.));
#32074=DIRECTION('center_axis',(-1.,0.,0.));
#32075=DIRECTION('ref_axis',(0.,-1.,0.));
#32076=DIRECTION('',(-0.38268343236509,0.923879532511287,1.1314261122877E-16));
#32077=DIRECTION('center_axis',(1.,0.,0.));
#32078=DIRECTION('ref_axis',(0.,0.,-1.));
#32079=DIRECTION('',(0.,0.,1.));
#32080=DIRECTION('center_axis',(1.,0.,0.));
#32081=DIRECTION('ref_axis',(0.,0.,-1.));
#32082=DIRECTION('',(0.,0.,-1.));
#32083=DIRECTION('',(0.,-1.,0.));
#32084=DIRECTION('center_axis',(0.707106781186548,-0.707106781186547,0.));
#32085=DIRECTION('ref_axis',(0.,0.,-1.));
#32086=DIRECTION('',(0.,0.,-1.));
#32087=DIRECTION('center_axis',(-0.707106781186548,0.707106781186547,0.));
#32088=DIRECTION('ref_axis',(0.707106781186547,0.707106781186548,0.));
#32089=DIRECTION('',(-0.577350269189608,-0.57735026918961,-0.57735026918966));
#32090=DIRECTION('center_axis',(0.707106781186554,0.707106781186541,0.));
#32091=DIRECTION('ref_axis',(0.,0.,-1.));
#32092=DIRECTION('center_axis',(-0.707106781186554,-0.707106781186541,0.));
#32093=DIRECTION('ref_axis',(-0.707106781186541,0.707106781186554,0.));
#32094=DIRECTION('',(0.,0.,1.));
#32095=DIRECTION('',(0.577350269189602,-0.577350269189613,0.577350269189663));
#32096=DIRECTION('center_axis',(0.707106781186579,0.,-0.707106781186516));
#32097=DIRECTION('ref_axis',(-0.707106781186516,0.,-0.707106781186579));
#32098=DIRECTION('',(0.,1.,0.));
#32099=DIRECTION('center_axis',(0.,0.,1.));
#32100=DIRECTION('ref_axis',(1.,0.,0.));
#32101=DIRECTION('',(1.,0.,0.));
#32102=DIRECTION('',(0.,-1.,0.));
#32103=DIRECTION('',(-1.,0.,0.));
#32104=DIRECTION('center_axis',(0.,-1.,0.));
#32105=DIRECTION('ref_axis',(-1.,0.,0.));
#32106=DIRECTION('',(1.,0.,0.));
#32107=DIRECTION('',(0.,0.,-1.));
#32108=DIRECTION('center_axis',(0.,1.,0.));
#32109=DIRECTION('ref_axis',(1.,0.,0.));
#32110=DIRECTION('',(0.,0.,-1.));
#32111=DIRECTION('',(-1.,0.,0.));
#32112=DIRECTION('center_axis',(1.,0.,0.));
#32113=DIRECTION('ref_axis',(0.,6.12323399573677E-17,-1.));
#32114=DIRECTION('center_axis',(1.,0.,0.));
#32115=DIRECTION('ref_axis',(0.,0.,-1.));
#32116=DIRECTION('center_axis',(0.,-0.707106781186547,0.707106781186548));
#32117=DIRECTION('ref_axis',(0.,0.707106781186548,0.707106781186547));
#32118=DIRECTION('',(-3.92313542605626E-18,-0.729395907617851,0.684091813976992));
#32119=DIRECTION('center_axis',(0.,0.707106781186548,0.707106781186547));
#32120=DIRECTION('ref_axis',(0.,0.707106781186548,-0.707106781186547));
#32121=DIRECTION('',(-3.92313542605626E-18,0.684091813976992,0.729395907617851));
#32122=DIRECTION('center_axis',(0.,0.707106781186547,-0.707106781186548));
#32123=DIRECTION('ref_axis',(0.,-0.707106781186546,-0.707106781186549));
#32124=DIRECTION('',(-3.92313542605623E-18,0.729395907617851,-0.684091813976992));
#32125=DIRECTION('center_axis',(0.,-0.707106781186547,-0.707106781186548));
#32126=DIRECTION('ref_axis',(0.,-0.707106781186548,0.707106781186547));
#32127=DIRECTION('',(-3.92313542605642E-18,-0.68409181397699,-0.729395907617853));
#32128=DIRECTION('center_axis',(1.,0.,0.));
#32129=DIRECTION('ref_axis',(0.,0.,-1.));
#32130=DIRECTION('center_axis',(0.,-1.,-1.22464679914735E-16));
#32131=DIRECTION('ref_axis',(0.,-1.22464679914735E-16,1.));
#32132=DIRECTION('center_axis',(-1.,0.,0.));
#32133=DIRECTION('ref_axis',(0.,0.,-1.));
#32134=DIRECTION('center_axis',(-1.,0.,0.));
#32135=DIRECTION('ref_axis',(0.,0.,-1.));
#32136=DIRECTION('center_axis',(-1.,0.,0.));
#32137=DIRECTION('ref_axis',(0.,0.,-1.));
#32138=DIRECTION('center_axis',(-1.,0.,0.));
#32139=DIRECTION('ref_axis',(0.,0.,-1.));
#32140=DIRECTION('center_axis',(-1.,0.,0.));
#32141=DIRECTION('ref_axis',(0.,0.,-1.));
#32142=DIRECTION('center_axis',(1.,0.,0.));
#32143=DIRECTION('ref_axis',(0.,1.,0.));
#32144=DIRECTION('center_axis',(1.,0.,0.));
#32145=DIRECTION('ref_axis',(0.,0.,-1.));
#32146=DIRECTION('',(-1.,0.,0.));
#32147=DIRECTION('center_axis',(1.,0.,0.));
#32148=DIRECTION('ref_axis',(0.,0.,-1.));
#49825=CARTESIAN_POINT('',(0.,0.,0.));
#49826=CARTESIAN_POINT('Origin',(4.89267766952966,0.,26.5));
#49827=CARTESIAN_POINT('',(4.93535533905933,2.46464466094067,26.5));
#49828=CARTESIAN_POINT('',(4.93535533905933,-2.46464466094067,26.5));
#49829=CARTESIAN_POINT('Origin',(4.93535533905933,0.,26.5));
#49830=CARTESIAN_POINT('Origin',(4.93535533905933,0.,26.5));
#49831=CARTESIAN_POINT('',(4.85,2.5,26.5));
#49832=CARTESIAN_POINT('',(4.89267766952966,2.48232233047034,26.5));
#49833=CARTESIAN_POINT('',(4.85,-2.5,26.5));
#49834=CARTESIAN_POINT('Origin',(4.85,0.,26.5));
#49835=CARTESIAN_POINT('Origin',(4.85,0.,26.5));
#49836=CARTESIAN_POINT('Origin',(2.9,0.,26.5));
#49837=CARTESIAN_POINT('',(0.95,-2.5,26.5));
#49838=CARTESIAN_POINT('',(2.9,-2.5,26.5));
#49839=CARTESIAN_POINT('',(0.95,2.5,26.5));
#49840=CARTESIAN_POINT('Origin',(0.95,0.,26.5));
#49841=CARTESIAN_POINT('Origin',(0.95,0.,26.5));
#49842=CARTESIAN_POINT('',(3.,2.28093439095105,25.4766045221046));
#49843=CARTESIAN_POINT('',(3.,1.0233954778954,24.219065609049));
#49844=CARTESIAN_POINT('Ctrl Pts',(3.,2.28093439095105,25.4766045221046));
#49845=CARTESIAN_POINT('Ctrl Pts',(2.88748169685465,2.28093439095105,25.4766045221046));
#49846=CARTESIAN_POINT('Ctrl Pts',(2.76831828254861,2.27115802886789,25.453965453567));
#49847=CARTESIAN_POINT('Ctrl Pts',(2.55048659094197,2.2289273827889,25.3667614364727));
#49848=CARTESIAN_POINT('Ctrl Pts',(2.45171547905721,2.19611046218737,25.3026299254791));
#49849=CARTESIAN_POINT('Ctrl Pts',(2.29613442646035,2.1138506187664,25.1627625092691));
#49850=CARTESIAN_POINT('Ctrl Pts',(2.22853784361638,2.05876256550245,25.0774506340239));
#49851=CARTESIAN_POINT('Ctrl Pts',(2.13845834389792,1.92557429855738,24.9017779820919));
#49852=CARTESIAN_POINT('Ctrl Pts',(2.11602564102564,1.8471621020331,24.8116281961004));
#49853=CARTESIAN_POINT('Ctrl Pts',(2.11602564102564,1.68837180389964,24.6528378979669));
#49854=CARTESIAN_POINT('Ctrl Pts',(2.13845834389792,1.59822201790808,24.5744257014426));
#49855=CARTESIAN_POINT('Ctrl Pts',(2.22853784361638,1.42254936597615,24.4412374344975));
#49856=CARTESIAN_POINT('Ctrl Pts',(2.29613442646035,1.33723749073094,24.3861493812336));
#49857=CARTESIAN_POINT('Ctrl Pts',(2.45171547905721,1.19737007452087,24.3038895378126));
#49858=CARTESIAN_POINT('Ctrl Pts',(2.55048659094197,1.1332385635273,24.2710726172111));
#49859=CARTESIAN_POINT('Ctrl Pts',(2.76831828254861,1.04603454643297,24.2288419711321));
#49860=CARTESIAN_POINT('Ctrl Pts',(2.88748169685465,1.0233954778954,24.219065609049));
#49861=CARTESIAN_POINT('Ctrl Pts',(3.,1.0233954778954,24.219065609049));
#49862=CARTESIAN_POINT('Ctrl Pts',(3.,1.0233954778954,24.2190656090489));
#49863=CARTESIAN_POINT('Ctrl Pts',(3.11251830314535,1.0233954778954,24.2190656090489));
#49864=CARTESIAN_POINT('Ctrl Pts',(3.23168171745139,1.04603454643297,24.2288419711321));
#49865=CARTESIAN_POINT('Ctrl Pts',(3.44951340905803,1.1332385635273,24.2710726172111));
#49866=CARTESIAN_POINT('Ctrl Pts',(3.54828452094279,1.19737007452087,24.3038895378126));
#49867=CARTESIAN_POINT('Ctrl Pts',(3.70386557353965,1.33723749073094,24.3861493812336));
#49868=CARTESIAN_POINT('Ctrl Pts',(3.77146215638362,1.42254936597615,24.4412374344975));
#49869=CARTESIAN_POINT('Ctrl Pts',(3.86154165610208,1.59822201790808,24.5744257014426));
#49870=CARTESIAN_POINT('Ctrl Pts',(3.88397435897436,1.68837180389964,24.6528378979669));
#49871=CARTESIAN_POINT('Ctrl Pts',(3.88397435897436,1.8471621020331,24.8116281961004));
#49872=CARTESIAN_POINT('Ctrl Pts',(3.86154165610208,1.92557429855738,24.9017779820919));
#49873=CARTESIAN_POINT('Ctrl Pts',(3.77146215638363,2.05876256550245,25.0774506340238));
#49874=CARTESIAN_POINT('Ctrl Pts',(3.70386557353965,2.1138506187664,25.1627625092691));
#49875=CARTESIAN_POINT('Ctrl Pts',(3.54828452094279,2.19611046218737,25.3026299254791));
#49876=CARTESIAN_POINT('Ctrl Pts',(3.44951340905803,2.2289273827889,25.3667614364727));
#49877=CARTESIAN_POINT('Ctrl Pts',(3.23168171745139,2.27115802886789,25.453965453567));
#49878=CARTESIAN_POINT('Ctrl Pts',(3.11251830314535,2.28093439095105,25.4766045221046));
#49879=CARTESIAN_POINT('Ctrl Pts',(3.,2.28093439095105,25.4766045221046));
#49880=CARTESIAN_POINT('',(3.,-1.0233954778954,24.219065609049));
#49881=CARTESIAN_POINT('',(3.,-2.28093439095105,25.4766045221046));
#49882=CARTESIAN_POINT('Ctrl Pts',(3.,-1.0233954778954,24.219065609049));
#49883=CARTESIAN_POINT('Ctrl Pts',(2.88748169685465,-1.0233954778954,24.219065609049));
#49884=CARTESIAN_POINT('Ctrl Pts',(2.76831828254861,-1.04603454643297,24.2288419711321));
#49885=CARTESIAN_POINT('Ctrl Pts',(2.55048659094197,-1.13323856352731,24.2710726172111));
#49886=CARTESIAN_POINT('Ctrl Pts',(2.45171547905721,-1.19737007452087,24.3038895378126));
#49887=CARTESIAN_POINT('Ctrl Pts',(2.29613442646035,-1.33723749073094,24.3861493812336));
#49888=CARTESIAN_POINT('Ctrl Pts',(2.22853784361638,-1.42254936597615,24.4412374344975));
#49889=CARTESIAN_POINT('Ctrl Pts',(2.13845834389792,-1.59822201790808,24.5744257014426));
#49890=CARTESIAN_POINT('Ctrl Pts',(2.11602564102564,-1.68837180389964,24.6528378979669));
#49891=CARTESIAN_POINT('Ctrl Pts',(2.11602564102564,-1.8471621020331,24.8116281961004));
#49892=CARTESIAN_POINT('Ctrl Pts',(2.13845834389792,-1.92557429855738,24.9017779820919));
#49893=CARTESIAN_POINT('Ctrl Pts',(2.22853784361637,-2.05876256550245,25.0774506340238));
#49894=CARTESIAN_POINT('Ctrl Pts',(2.29613442646035,-2.1138506187664,25.1627625092691));
#49895=CARTESIAN_POINT('Ctrl Pts',(2.45171547905721,-2.19611046218737,25.3026299254791));
#49896=CARTESIAN_POINT('Ctrl Pts',(2.55048659094197,-2.2289273827889,25.3667614364727));
#49897=CARTESIAN_POINT('Ctrl Pts',(2.76831828254861,-2.27115802886789,25.453965453567));
#49898=CARTESIAN_POINT('Ctrl Pts',(2.88748169685465,-2.28093439095105,25.4766045221046));
#49899=CARTESIAN_POINT('Ctrl Pts',(3.,-2.28093439095105,25.4766045221046));
#49900=CARTESIAN_POINT('Ctrl Pts',(3.,-2.28093439095105,25.4766045221046));
#49901=CARTESIAN_POINT('Ctrl Pts',(3.11251830314535,-2.28093439095105,25.4766045221046));
#49902=CARTESIAN_POINT('Ctrl Pts',(3.23168171745139,-2.27115802886789,25.453965453567));
#49903=CARTESIAN_POINT('Ctrl Pts',(3.44951340905803,-2.2289273827889,25.3667614364727));
#49904=CARTESIAN_POINT('Ctrl Pts',(3.54828452094279,-2.19611046218737,25.3026299254791));
#49905=CARTESIAN_POINT('Ctrl Pts',(3.70386557353965,-2.1138506187664,25.1627625092691));
#49906=CARTESIAN_POINT('Ctrl Pts',(3.77146215638363,-2.05876256550245,25.0774506340238));
#49907=CARTESIAN_POINT('Ctrl Pts',(3.86154165610208,-1.92557429855738,24.9017779820919));
#49908=CARTESIAN_POINT('Ctrl Pts',(3.88397435897436,-1.8471621020331,24.8116281961004));
#49909=CARTESIAN_POINT('Ctrl Pts',(3.88397435897436,-1.68837180389964,24.6528378979669));
#49910=CARTESIAN_POINT('Ctrl Pts',(3.86154165610208,-1.59822201790809,24.5744257014426));
#49911=CARTESIAN_POINT('Ctrl Pts',(3.77146215638363,-1.42254936597616,24.4412374344975));
#49912=CARTESIAN_POINT('Ctrl Pts',(3.70386557353965,-1.33723749073094,24.3861493812336));
#49913=CARTESIAN_POINT('Ctrl Pts',(3.54828452094279,-1.19737007452087,24.3038895378126));
#49914=CARTESIAN_POINT('Ctrl Pts',(3.44951340905803,-1.13323856352731,24.2710726172111));
#49915=CARTESIAN_POINT('Ctrl Pts',(3.23168171745139,-1.04603454643297,24.2288419711321));
#49916=CARTESIAN_POINT('Ctrl Pts',(3.11251830314535,-1.0233954778954,24.219065609049));
#49917=CARTESIAN_POINT('Ctrl Pts',(3.,-1.0233954778954,24.219065609049));
#49918=CARTESIAN_POINT('',(3.,-2.28093439095105,27.5233954778954));
#49919=CARTESIAN_POINT('',(3.,-1.0233954778954,28.7809343909511));
#49920=CARTESIAN_POINT('Ctrl Pts',(3.,-2.28093439095105,27.5233954778954));
#49921=CARTESIAN_POINT('Ctrl Pts',(2.88748169685465,-2.28093439095105,27.5233954778954));
#49922=CARTESIAN_POINT('Ctrl Pts',(2.76831828254861,-2.27115802886789,27.546034546433));
#49923=CARTESIAN_POINT('Ctrl Pts',(2.55048659094197,-2.2289273827889,27.6332385635273));
#49924=CARTESIAN_POINT('Ctrl Pts',(2.45171547905721,-2.19611046218737,27.6973700745209));
#49925=CARTESIAN_POINT('Ctrl Pts',(2.29613442646035,-2.1138506187664,27.8372374907309));
#49926=CARTESIAN_POINT('Ctrl Pts',(2.22853784361637,-2.05876256550245,27.9225493659762));
#49927=CARTESIAN_POINT('Ctrl Pts',(2.13845834389792,-1.92557429855738,28.0982220179081));
#49928=CARTESIAN_POINT('Ctrl Pts',(2.11602564102564,-1.8471621020331,28.1883718038996));
#49929=CARTESIAN_POINT('Ctrl Pts',(2.11602564102564,-1.68837180389964,28.3471621020331));
#49930=CARTESIAN_POINT('Ctrl Pts',(2.13845834389792,-1.59822201790808,28.4255742985574));
#49931=CARTESIAN_POINT('Ctrl Pts',(2.22853784361637,-1.42254936597615,28.5587625655025));
#49932=CARTESIAN_POINT('Ctrl Pts',(2.29613442646035,-1.33723749073094,28.6138506187664));
#49933=CARTESIAN_POINT('Ctrl Pts',(2.45171547905721,-1.19737007452087,28.6961104621874));
#49934=CARTESIAN_POINT('Ctrl Pts',(2.55048659094197,-1.13323856352731,28.7289273827889));
#49935=CARTESIAN_POINT('Ctrl Pts',(2.76831828254861,-1.04603454643297,28.7711580288679));
#49936=CARTESIAN_POINT('Ctrl Pts',(2.88748169685465,-1.0233954778954,28.7809343909511));
#49937=CARTESIAN_POINT('Ctrl Pts',(3.,-1.0233954778954,28.7809343909511));
#49938=CARTESIAN_POINT('Ctrl Pts',(3.,-1.0233954778954,28.7809343909511));
#49939=CARTESIAN_POINT('Ctrl Pts',(3.11251830314535,-1.0233954778954,28.7809343909511));
#49940=CARTESIAN_POINT('Ctrl Pts',(3.23168171745139,-1.04603454643297,28.7711580288679));
#49941=CARTESIAN_POINT('Ctrl Pts',(3.44951340905803,-1.13323856352731,28.7289273827889));
#49942=CARTESIAN_POINT('Ctrl Pts',(3.54828452094279,-1.19737007452087,28.6961104621874));
#49943=CARTESIAN_POINT('Ctrl Pts',(3.70386557353965,-1.33723749073094,28.6138506187664));
#49944=CARTESIAN_POINT('Ctrl Pts',(3.77146215638363,-1.42254936597615,28.5587625655025));
#49945=CARTESIAN_POINT('Ctrl Pts',(3.86154165610208,-1.59822201790808,28.4255742985574));
#49946=CARTESIAN_POINT('Ctrl Pts',(3.88397435897436,-1.68837180389964,28.3471621020331));
#49947=CARTESIAN_POINT('Ctrl Pts',(3.88397435897436,-1.8471621020331,28.1883718038996));
#49948=CARTESIAN_POINT('Ctrl Pts',(3.86154165610208,-1.92557429855738,28.0982220179081));
#49949=CARTESIAN_POINT('Ctrl Pts',(3.77146215638362,-2.05876256550245,27.9225493659761));
#49950=CARTESIAN_POINT('Ctrl Pts',(3.70386557353965,-2.1138506187664,27.8372374907309));
#49951=CARTESIAN_POINT('Ctrl Pts',(3.54828452094279,-2.19611046218737,27.6973700745209));
#49952=CARTESIAN_POINT('Ctrl Pts',(3.44951340905803,-2.2289273827889,27.6332385635273));
#49953=CARTESIAN_POINT('Ctrl Pts',(3.23168171745139,-2.27115802886789,27.546034546433));
#49954=CARTESIAN_POINT('Ctrl Pts',(3.11251830314535,-2.28093439095105,27.5233954778954));
#49955=CARTESIAN_POINT('Ctrl Pts',(3.,-2.28093439095105,27.5233954778954));
#49956=CARTESIAN_POINT('',(3.,1.0233954778954,28.780934390951));
#49957=CARTESIAN_POINT('',(3.,2.28093439095105,27.5233954778954));
#49958=CARTESIAN_POINT('Ctrl Pts',(3.,1.0233954778954,28.780934390951));
#49959=CARTESIAN_POINT('Ctrl Pts',(2.88748169685465,1.0233954778954,28.780934390951));
#49960=CARTESIAN_POINT('Ctrl Pts',(2.76831828254861,1.04603454643297,28.7711580288679));
#49961=CARTESIAN_POINT('Ctrl Pts',(2.55048659094197,1.13323856352731,28.7289273827889));
#49962=CARTESIAN_POINT('Ctrl Pts',(2.45171547905721,1.19737007452087,28.6961104621874));
#49963=CARTESIAN_POINT('Ctrl Pts',(2.29613442646035,1.33723749073094,28.6138506187664));
#49964=CARTESIAN_POINT('Ctrl Pts',(2.22853784361638,1.42254936597615,28.5587625655025));
#49965=CARTESIAN_POINT('Ctrl Pts',(2.13845834389792,1.59822201790808,28.4255742985574));
#49966=CARTESIAN_POINT('Ctrl Pts',(2.11602564102564,1.68837180389964,28.3471621020331));
#49967=CARTESIAN_POINT('Ctrl Pts',(2.11602564102564,1.8471621020331,28.1883718038996));
#49968=CARTESIAN_POINT('Ctrl Pts',(2.13845834389792,1.92557429855738,28.0982220179081));
#49969=CARTESIAN_POINT('Ctrl Pts',(2.22853784361637,2.05876256550245,27.9225493659761));
#49970=CARTESIAN_POINT('Ctrl Pts',(2.29613442646034,2.1138506187664,27.8372374907309));
#49971=CARTESIAN_POINT('Ctrl Pts',(2.45171547905721,2.19611046218737,27.6973700745209));
#49972=CARTESIAN_POINT('Ctrl Pts',(2.55048659094197,2.2289273827889,27.6332385635273));
#49973=CARTESIAN_POINT('Ctrl Pts',(2.76831828254861,2.27115802886789,27.546034546433));
#49974=CARTESIAN_POINT('Ctrl Pts',(2.88748169685465,2.28093439095105,27.5233954778954));
#49975=CARTESIAN_POINT('Ctrl Pts',(3.,2.28093439095105,27.5233954778954));
#49976=CARTESIAN_POINT('Ctrl Pts',(3.,2.28093439095105,27.5233954778954));
#49977=CARTESIAN_POINT('Ctrl Pts',(3.11251830314535,2.28093439095105,27.5233954778954));
#49978=CARTESIAN_POINT('Ctrl Pts',(3.23168171745139,2.27115802886789,27.546034546433));
#49979=CARTESIAN_POINT('Ctrl Pts',(3.44951340905803,2.2289273827889,27.6332385635273));
#49980=CARTESIAN_POINT('Ctrl Pts',(3.54828452094279,2.19611046218737,27.6973700745209));
#49981=CARTESIAN_POINT('Ctrl Pts',(3.70386557353965,2.1138506187664,27.8372374907309));
#49982=CARTESIAN_POINT('Ctrl Pts',(3.77146215638363,2.05876256550245,27.9225493659761));
#49983=CARTESIAN_POINT('Ctrl Pts',(3.86154165610208,1.92557429855738,28.0982220179081));
#49984=CARTESIAN_POINT('Ctrl Pts',(3.88397435897436,1.8471621020331,28.1883718038996));
#49985=CARTESIAN_POINT('Ctrl Pts',(3.88397435897436,1.68837180389964,28.3471621020331));
#49986=CARTESIAN_POINT('Ctrl Pts',(3.86154165610208,1.59822201790808,28.4255742985574));
#49987=CARTESIAN_POINT('Ctrl Pts',(3.77146215638362,1.42254936597615,28.5587625655025));
#49988=CARTESIAN_POINT('Ctrl Pts',(3.70386557353965,1.33723749073094,28.6138506187664));
#49989=CARTESIAN_POINT('Ctrl Pts',(3.54828452094279,1.19737007452087,28.6961104621874));
#49990=CARTESIAN_POINT('Ctrl Pts',(3.44951340905803,1.13323856352731,28.7289273827889));
#49991=CARTESIAN_POINT('Ctrl Pts',(3.23168171745139,1.04603454643297,28.7711580288679));
#49992=CARTESIAN_POINT('Ctrl Pts',(3.11251830314535,1.0233954778954,28.780934390951));
#49993=CARTESIAN_POINT('Ctrl Pts',(3.,1.0233954778954,28.780934390951));
#49994=CARTESIAN_POINT('Origin',(4.95,0.,26.5));
#49995=CARTESIAN_POINT('',(4.96464466094067,2.43535533905933,26.5));
#49996=CARTESIAN_POINT('',(4.96464466094067,-2.43535533905933,26.5));
#49997=CARTESIAN_POINT('Origin',(4.96464466094067,0.,26.5));
#49998=CARTESIAN_POINT('Origin',(4.96464466094067,0.,26.5));
#49999=CARTESIAN_POINT('',(4.95,-2.45,26.5));
#50000=CARTESIAN_POINT('Origin',(0.907322330470336,0.,26.5));
#50001=CARTESIAN_POINT('',(0.864644660940672,2.46464466094067,26.5));
#50002=CARTESIAN_POINT('',(0.907322330470336,2.48232233047034,26.5));
#50003=CARTESIAN_POINT('',(0.864644660940673,-2.46464466094067,26.5));
#50004=CARTESIAN_POINT('Origin',(0.864644660940672,0.,26.5));
#50005=CARTESIAN_POINT('Origin',(0.864644660940672,0.,26.5));
#50006=CARTESIAN_POINT('Origin',(0.85,0.,26.5));
#50007=CARTESIAN_POINT('',(0.835355339059327,-2.43535533905933,26.5));
#50008=CARTESIAN_POINT('',(0.85,-2.45,26.5));
#50009=CARTESIAN_POINT('',(0.835355339059327,2.43535533905933,26.5));
#50010=CARTESIAN_POINT('Origin',(0.835355339059327,0.,26.5));
#50011=CARTESIAN_POINT('Origin',(0.835355339059327,0.,26.5));
#50012=CARTESIAN_POINT('Origin',(0.817677669529664,0.,26.5));
#50013=CARTESIAN_POINT('',(0.8,2.35,26.5));
#50014=CARTESIAN_POINT('',(0.817677669529664,2.39267766952966,26.5));
#50015=CARTESIAN_POINT('Origin',(0.8,0.,26.5));
#50016=CARTESIAN_POINT('Origin',(0.8,2.4,26.5));
#50017=CARTESIAN_POINT('',(0.8,-0.46,26.5));
#50018=CARTESIAN_POINT('Origin',(0.8,0.,26.5));
#50019=CARTESIAN_POINT('Origin',(4.98232233047034,0.,26.5));
#50020=CARTESIAN_POINT('',(5.,2.35,26.5));
#50021=CARTESIAN_POINT('Origin',(5.,0.,26.5));
#50022=CARTESIAN_POINT('',(4.98232233047034,2.39267766952966,26.5));
#50023=CARTESIAN_POINT('Origin',(5.,1.,26.5));
#50024=CARTESIAN_POINT('',(5.,0.3025,27.453149384934));
#50025=CARTESIAN_POINT('',(5.,0.3025,27.78));
#50026=CARTESIAN_POINT('',(5.,0.3025,27.115));
#50027=CARTESIAN_POINT('',(5.,-0.3025,27.453149384934));
#50028=CARTESIAN_POINT('Origin',(5.,0.,26.5));
#50029=CARTESIAN_POINT('',(5.,-0.3025,27.78));
#50030=CARTESIAN_POINT('',(5.,-0.3025,27.115));
#50031=CARTESIAN_POINT('',(5.,0.5,27.78));
#50032=CARTESIAN_POINT('Origin',(4.975,0.2775,27.115));
#50033=CARTESIAN_POINT('',(4.95,0.2525,27.73));
#50034=CARTESIAN_POINT('',(4.95,0.2525,27.4675968943729));
#50035=CARTESIAN_POINT('',(4.95,0.2525,27.115));
#50036=CARTESIAN_POINT('Origin',(4.6975,0.,26.5));
#50037=CARTESIAN_POINT('',(5.,0.3025,27.78));
#50038=CARTESIAN_POINT('Origin',(4.975,-0.2775,27.115));
#50039=CARTESIAN_POINT('',(4.95,-0.2525,27.4675968943729));
#50040=CARTESIAN_POINT('Origin',(4.69750000000001,0.,26.5));
#50041=CARTESIAN_POINT('',(4.95,-0.2525,27.73));
#50042=CARTESIAN_POINT('',(4.95,-0.2525,27.115));
#50043=CARTESIAN_POINT('',(4.95,-0.2525,27.73));
#50044=CARTESIAN_POINT('Origin',(4.975,0.5,27.755));
#50045=CARTESIAN_POINT('',(4.95,0.5,27.73));
#50046=CARTESIAN_POINT('Origin',(3.2,0.,27.73));
#50047=CARTESIAN_POINT('',(1.3,-0.2525,27.73));
#50048=CARTESIAN_POINT('',(1.3,-0.2525,27.73));
#50049=CARTESIAN_POINT('',(1.3,0.2525,27.73));
#50050=CARTESIAN_POINT('',(1.3,0.2525,27.73));
#50051=CARTESIAN_POINT('',(5.1,0.2525,27.73));
#50052=CARTESIAN_POINT('Origin',(5.1,-0.2525,27.73));
#50053=CARTESIAN_POINT('',(1.3,-0.2525,27.4675968943729));
#50054=CARTESIAN_POINT('',(3.15,-0.2525,27.4675968943729));
#50055=CARTESIAN_POINT('',(1.3,-0.2525,27.73));
#50056=CARTESIAN_POINT('Origin',(1.3,0.2525,27.73));
#50057=CARTESIAN_POINT('',(1.3,0.2525,27.4675968943729));
#50058=CARTESIAN_POINT('',(1.3,0.2525,27.73));
#50059=CARTESIAN_POINT('',(3.15,0.2525,27.4675968943729));
#50060=CARTESIAN_POINT('Origin',(3.15,0.,26.5));
#50061=CARTESIAN_POINT('Origin',(1.3,0.,26.5));
#50062=CARTESIAN_POINT('Origin',(3.,4.17193000900063,22.3280699909994));
#50063=CARTESIAN_POINT('',(3.65899840720328,6.73112601132474,19.7688739886753));
#50064=CARTESIAN_POINT('',(3.,6.08767497843372,19.4693376302832));
#50065=CARTESIAN_POINT('Ctrl Pts',(3.65899840720328,6.73112601132474,19.7688739886753));
#50066=CARTESIAN_POINT('Ctrl Pts',(3.65899840720328,6.72679268575653,19.764540663107));
#50067=CARTESIAN_POINT('Ctrl Pts',(3.65891512098012,6.72241218185797,19.7602566839318));
#50068=CARTESIAN_POINT('Ctrl Pts',(3.65781547543884,6.69317457331001,19.7322924236316));
#50069=CARTESIAN_POINT('Ctrl Pts',(3.65428413830508,6.66710502404872,19.7103330586802));
#50070=CARTESIAN_POINT('Ctrl Pts',(3.63870034113718,6.59727918356102,19.6581255858253));
#50071=CARTESIAN_POINT('Ctrl Pts',(3.62306713231032,6.55278988756777,19.6310282895777));
#50072=CARTESIAN_POINT('Ctrl Pts',(3.56551968033953,6.43088892463072,19.5676842688384));
#50073=CARTESIAN_POINT('Ctrl Pts',(3.51273077708496,6.3539988734894,19.53969222603));
#50074=CARTESIAN_POINT('Ctrl Pts',(3.3884774805394,6.2283829770698,19.5010021486756));
#50075=CARTESIAN_POINT('Ctrl Pts',(3.3188912623837,6.1772205194954,19.4887543145494));
#50076=CARTESIAN_POINT('Ctrl Pts',(3.17532557849005,6.11134378631976,19.4739796943783));
#50077=CARTESIAN_POINT('Ctrl Pts',(3.10504775292283,6.09288250834592,19.4703811570922));
#50078=CARTESIAN_POINT('Ctrl Pts',(3.02160267663661,6.08799029722494,19.4694006361368));
#50079=CARTESIAN_POINT('Ctrl Pts',(3.01078870740022,6.08767497843372,19.4693376302832));
#50080=CARTESIAN_POINT('Ctrl Pts',(3.,6.08767497843372,19.4693376302832));
#50081=CARTESIAN_POINT('',(3.,7.03066236971681,20.4123250215663));
#50082=CARTESIAN_POINT('Ctrl Pts',(3.,7.03066236971681,20.4123250215663));
#50083=CARTESIAN_POINT('Ctrl Pts',(3.01771871221482,7.03066236971681,20.4123250215663));
#50084=CARTESIAN_POINT('Ctrl Pts',(3.03548526784966,7.03049271525968,20.4114744757539));
#50085=CARTESIAN_POINT('Ctrl Pts',(3.12997701049201,7.02866026735908,20.4023629263842));
#50086=CARTESIAN_POINT('Ctrl Pts',(3.20348422043859,7.02410185118279,20.379195333342));
#50087=CARTESIAN_POINT('Ctrl Pts',(3.34957484663758,7.00637212768387,20.3026046352004));
#50088=CARTESIAN_POINT('Ctrl Pts',(3.41865686125493,6.99216527474278,20.2459676889049));
#50089=CARTESIAN_POINT('Ctrl Pts',(3.53708659094303,6.94832361568055,20.1129667523922));
#50090=CARTESIAN_POINT('Ctrl Pts',(3.5854928838657,6.91741798080179,20.0347556209823));
#50091=CARTESIAN_POINT('Ctrl Pts',(3.6332576564077,6.8511743356788,19.9182014933262));
#50092=CARTESIAN_POINT('Ctrl Pts',(3.64497180237219,6.82563598060614,19.879439709583));
#50093=CARTESIAN_POINT('Ctrl Pts',(3.65660045499355,6.77613678192328,19.8166848017198));
#50094=CARTESIAN_POINT('Ctrl Pts',(3.65899840720328,6.75441124717323,19.7921592245237));
#50095=CARTESIAN_POINT('Ctrl Pts',(3.65899840720328,6.73112601132474,19.7688739886753));
#50096=CARTESIAN_POINT('Ctrl Pts',(3.,6.08767497843372,19.4693376302832));
#50097=CARTESIAN_POINT('Ctrl Pts',(2.93740375632011,6.08767497843372,19.4693376302832));
#50098=CARTESIAN_POINT('Ctrl Pts',(2.87565789134425,6.09830402968064,19.4713955392217));
#50099=CARTESIAN_POINT('Ctrl Pts',(2.73401545070695,6.14671873130702,19.4817369535417));
#50100=CARTESIAN_POINT('Ctrl Pts',(2.65923300361176,6.19233182892452,19.4918543552589));
#50101=CARTESIAN_POINT('Ctrl Pts',(2.52172868443338,6.31191640618337,19.525619137228));
#50102=CARTESIAN_POINT('Ctrl Pts',(2.46172409835092,6.38885879373983,19.5508628055546));
#50103=CARTESIAN_POINT('Ctrl Pts',(2.39060701245704,6.51897766283336,19.6119448626741));
#50104=CARTESIAN_POINT('Ctrl Pts',(2.36956327353234,6.57078939327557,19.6407922394961));
#50105=CARTESIAN_POINT('Ctrl Pts',(2.34883638351778,6.64971896474124,19.6965382745686));
#50106=CARTESIAN_POINT('Ctrl Pts',(2.34397532261961,6.67778206838811,19.7189689436771));
#50107=CARTESIAN_POINT('Ctrl Pts',(2.34028669329881,6.72781049660135,19.7647333834671));
#50108=CARTESIAN_POINT('Ctrl Pts',(2.34077606978153,6.74979295500866,19.7872890495768));
#50109=CARTESIAN_POINT('Ctrl Pts',(2.34680248319783,6.79615911042744,19.8405985114576));
#50110=CARTESIAN_POINT('Ctrl Pts',(2.35349632945342,6.81939902656569,19.8715417922134));
#50111=CARTESIAN_POINT('Ctrl Pts',(2.38103390803266,6.87804712505273,19.9605120359057));
#50112=CARTESIAN_POINT('Ctrl Pts',(2.40863932166359,6.90772580028368,20.0194824078591));
#50113=CARTESIAN_POINT('Ctrl Pts',(2.49309498094617,6.96395620747032,20.1528861413115));
#50114=CARTESIAN_POINT('Ctrl Pts',(2.55769731566219,6.9858385252213,20.2258560176688));
#50115=CARTESIAN_POINT('Ctrl Pts',(2.69643706868986,7.01339895805737,20.3305435155435));
#50116=CARTESIAN_POINT('Ctrl Pts',(2.76629587634974,7.02135172130659,20.3674349512207));
#50117=CARTESIAN_POINT('Ctrl Pts',(2.89345183041008,7.02914761950448,20.404565188633));
#50118=CARTESIAN_POINT('Ctrl Pts',(2.94650789475061,7.03066236971681,20.4123250215663));
#50119=CARTESIAN_POINT('Ctrl Pts',(3.,7.03066236971681,20.4123250215663));
#50120=CARTESIAN_POINT('',(3.,3.62392225358105,21.7800622355798));
#50121=CARTESIAN_POINT('Origin',(3.,-4.17193000900063,22.3280699909994));
#50122=CARTESIAN_POINT('',(3.65899840720328,-6.73112601132475,19.7688739886753));
#50123=CARTESIAN_POINT('',(3.,-7.03066236971681,20.4123250215663));
#50124=CARTESIAN_POINT('Ctrl Pts',(3.65899840720328,-6.73112601132475,19.7688739886753));
#50125=CARTESIAN_POINT('Ctrl Pts',(3.65899840720328,-6.73545933689293,19.7732073142435));
#50126=CARTESIAN_POINT('Ctrl Pts',(3.65891512098013,-6.73974331606821,19.777587818142));
#50127=CARTESIAN_POINT('Ctrl Pts',(3.65781547543884,-6.76770757636838,19.80682542669));
#50128=CARTESIAN_POINT('Ctrl Pts',(3.65428413830508,-6.78966694131985,19.8328949759513));
#50129=CARTESIAN_POINT('Ctrl Pts',(3.63870034113718,-6.84187441417476,19.902720816439));
#50130=CARTESIAN_POINT('Ctrl Pts',(3.6230671323103,-6.86897171042233,19.9472101124323));
#50131=CARTESIAN_POINT('Ctrl Pts',(3.56551968033951,-6.93231573116165,20.0691110753693));
#50132=CARTESIAN_POINT('Ctrl Pts',(3.51273077708492,-6.96030777396999,20.1460011265106));
#50133=CARTESIAN_POINT('Ctrl Pts',(3.38847748053938,-6.99899785132438,20.2716170229302));
#50134=CARTESIAN_POINT('Ctrl Pts',(3.31889126238367,-7.0112456854506,20.3227794805046));
#50135=CARTESIAN_POINT('Ctrl Pts',(3.17532557849002,-7.02602030562166,20.3886562136803));
#50136=CARTESIAN_POINT('Ctrl Pts',(3.10504775292279,-7.0296188429078,20.4071174916541));
#50137=CARTESIAN_POINT('Ctrl Pts',(3.0216026766366,-7.03059936386324,20.4120097027751));
#50138=CARTESIAN_POINT('Ctrl Pts',(3.01078870740021,-7.03066236971681,20.4123250215663));
#50139=CARTESIAN_POINT('Ctrl Pts',(3.,-7.03066236971681,20.4123250215663));
#50140=CARTESIAN_POINT('',(3.,-6.08767497843373,19.4693376302832));
#50141=CARTESIAN_POINT('Ctrl Pts',(3.,-6.08767497843373,19.4693376302832));
#50142=CARTESIAN_POINT('Ctrl Pts',(3.01771871221484,-6.08767497843373,19.4693376302832));
#50143=CARTESIAN_POINT('Ctrl Pts',(3.03548526784968,-6.08852552424608,19.4695072847403));
#50144=CARTESIAN_POINT('Ctrl Pts',(3.12997701049206,-6.09763707361583,19.4713397326409));
#50145=CARTESIAN_POINT('Ctrl Pts',(3.20348422043864,-6.12080466665799,19.4758981488172));
#50146=CARTESIAN_POINT('Ctrl Pts',(3.34957484663764,-6.19739536479959,19.4936278723161));
#50147=CARTESIAN_POINT('Ctrl Pts',(3.41865686125498,-6.25403231109519,19.5078347252572));
#50148=CARTESIAN_POINT('Ctrl Pts',(3.53708659094306,-6.38703324760786,19.5516763843195));
#50149=CARTESIAN_POINT('Ctrl Pts',(3.58549288386572,-6.46524437901772,19.5825820191982));
#50150=CARTESIAN_POINT('Ctrl Pts',(3.63325765640772,-6.58179850667387,19.6488256643212));
#50151=CARTESIAN_POINT('Ctrl Pts',(3.64497180237219,-6.62056029041704,19.6743640193939));
#50152=CARTESIAN_POINT('Ctrl Pts',(3.65660045499355,-6.68331519828019,19.7238632180767));
#50153=CARTESIAN_POINT('Ctrl Pts',(3.65899840720328,-6.70784077547626,19.7455887528268));
#50154=CARTESIAN_POINT('Ctrl Pts',(3.65899840720328,-6.73112601132475,19.7688739886753));
#50155=CARTESIAN_POINT('Ctrl Pts',(3.,-7.03066236971681,20.4123250215663));
#50156=CARTESIAN_POINT('Ctrl Pts',(2.93740375632008,-7.03066236971681,20.4123250215663));
#50157=CARTESIAN_POINT('Ctrl Pts',(2.87565789134422,-7.02860446077828,20.4016959703194));
#50158=CARTESIAN_POINT('Ctrl Pts',(2.73401545070689,-7.01826304645833,20.353281268693));
#50159=CARTESIAN_POINT('Ctrl Pts',(2.6592330036117,-7.00814564474112,20.3076681710754));
#50160=CARTESIAN_POINT('Ctrl Pts',(2.52172868443334,-6.97438086277199,20.1880835938166));
#50161=CARTESIAN_POINT('Ctrl Pts',(2.46172409835089,-6.94913719444542,20.1111412062601));
#50162=CARTESIAN_POINT('Ctrl Pts',(2.39060701245703,-6.88805513732593,19.9810223371666));
#50163=CARTESIAN_POINT('Ctrl Pts',(2.36956327353233,-6.85920776050386,19.9292106067244));
#50164=CARTESIAN_POINT('Ctrl Pts',(2.34883638351777,-6.80346172543135,19.8502810352587));
#50165=CARTESIAN_POINT('Ctrl Pts',(2.34397532261961,-6.78103105632287,19.8222179316119));
#50166=CARTESIAN_POINT('Ctrl Pts',(2.34028669329881,-6.73526661653286,19.7721895033986));
#50167=CARTESIAN_POINT('Ctrl Pts',(2.34077606978153,-6.71271095042321,19.7502070449913));
#50168=CARTESIAN_POINT('Ctrl Pts',(2.34680248319783,-6.65940148854232,19.7038408895725));
#50169=CARTESIAN_POINT('Ctrl Pts',(2.35349632945343,-6.62845820778657,19.6806009734343));
#50170=CARTESIAN_POINT('Ctrl Pts',(2.38103390803267,-6.53948796409423,19.6219528749472));
#50171=CARTESIAN_POINT('Ctrl Pts',(2.40863932166361,-6.48051759214088,19.5922741997163));
#50172=CARTESIAN_POINT('Ctrl Pts',(2.49309498094621,-6.34711385868844,19.5360437925297));
#50173=CARTESIAN_POINT('Ctrl Pts',(2.55769731566224,-6.2741439823312,19.5141614747787));
#50174=CARTESIAN_POINT('Ctrl Pts',(2.6964370686899,-6.16945648445649,19.4866010419426));
#50175=CARTESIAN_POINT('Ctrl Pts',(2.76629587634979,-6.13256504877927,19.4786482786934));
#50176=CARTESIAN_POINT('Ctrl Pts',(2.89345183041011,-6.09543481136695,19.4708523804955));
#50177=CARTESIAN_POINT('Ctrl Pts',(2.94650789475063,-6.08767497843372,19.4693376302832));
#50178=CARTESIAN_POINT('Ctrl Pts',(3.,-6.08767497843372,19.4693376302832));
#50179=CARTESIAN_POINT('',(3.,-4.71993776442021,22.8760777464189));
#50180=CARTESIAN_POINT('Origin',(3.,-4.17193000900063,30.6719300090006));
#50181=CARTESIAN_POINT('',(3.65899840720328,-6.73112601132474,33.2311260113247));
#50182=CARTESIAN_POINT('',(3.,-6.08767497843372,33.5306623697168));
#50183=CARTESIAN_POINT('Ctrl Pts',(3.65899840720328,-6.73112601132474,33.2311260113247));
#50184=CARTESIAN_POINT('Ctrl Pts',(3.65899840720328,-6.72679268575659,33.2354593368929));
#50185=CARTESIAN_POINT('Ctrl Pts',(3.65891512098013,-6.72241218185809,33.2397433160682));
#50186=CARTESIAN_POINT('Ctrl Pts',(3.65781547543884,-6.69317457330999,33.2677075763684));
#50187=CARTESIAN_POINT('Ctrl Pts',(3.65428413830508,-6.6671050240487,33.2896669413199));
#50188=CARTESIAN_POINT('Ctrl Pts',(3.63870034113717,-6.59727918356096,33.3418744141748));
#50189=CARTESIAN_POINT('Ctrl Pts',(3.62306713231028,-6.55278988756768,33.3689717104224));
#50190=CARTESIAN_POINT('Ctrl Pts',(3.5655196803395,-6.43088892463065,33.4323157311617));
#50191=CARTESIAN_POINT('Ctrl Pts',(3.51273077708491,-6.35399887348934,33.46030777397));
#50192=CARTESIAN_POINT('Ctrl Pts',(3.38847748053935,-6.22838297706974,33.4989978513244));
#50193=CARTESIAN_POINT('Ctrl Pts',(3.31889126238363,-6.17722051949536,33.5112456854506));
#50194=CARTESIAN_POINT('Ctrl Pts',(3.17532557849001,-6.11134378631973,33.5260203056217));
#50195=CARTESIAN_POINT('Ctrl Pts',(3.10504775292278,-6.09288250834591,33.5296188429078));
#50196=CARTESIAN_POINT('Ctrl Pts',(3.02160267663661,-6.08799029722494,33.5305993638632));
#50197=CARTESIAN_POINT('Ctrl Pts',(3.01078870740022,-6.08767497843372,33.5306623697168));
#50198=CARTESIAN_POINT('Ctrl Pts',(3.,-6.08767497843372,33.5306623697168));
#50199=CARTESIAN_POINT('',(3.,-7.03066236971681,32.5876749784337));
#50200=CARTESIAN_POINT('Ctrl Pts',(3.,-7.03066236971681,32.5876749784337));
#50201=CARTESIAN_POINT('Ctrl Pts',(3.01771871221484,-7.03066236971681,32.5876749784337));
#50202=CARTESIAN_POINT('Ctrl Pts',(3.03548526784969,-7.03049271525968,32.5885255242461));
#50203=CARTESIAN_POINT('Ctrl Pts',(3.1299770104921,-7.02866026735908,32.5976370736158));
#50204=CARTESIAN_POINT('Ctrl Pts',(3.20348422043866,-7.02410185118278,32.620804666658));
#50205=CARTESIAN_POINT('Ctrl Pts',(3.34957484663769,-7.00637212768386,32.6973953647996));
#50206=CARTESIAN_POINT('Ctrl Pts',(3.41865686125501,-6.99216527474276,32.7540323110952));
#50207=CARTESIAN_POINT('Ctrl Pts',(3.53708659094313,-6.94832361568051,32.8870332476079));
#50208=CARTESIAN_POINT('Ctrl Pts',(3.58549288386575,-6.91741798080174,32.9652443790178));
#50209=CARTESIAN_POINT('Ctrl Pts',(3.63325765640772,-6.85117433567877,33.0817985066739));
#50210=CARTESIAN_POINT('Ctrl Pts',(3.6449718023722,-6.8256359806061,33.1205602904171));
#50211=CARTESIAN_POINT('Ctrl Pts',(3.65660045499355,-6.77613678192326,33.1833151982802));
#50212=CARTESIAN_POINT('Ctrl Pts',(3.65899840720328,-6.75441124717321,33.2078407754763));
#50213=CARTESIAN_POINT('Ctrl Pts',(3.65899840720328,-6.73112601132474,33.2311260113247));
#50214=CARTESIAN_POINT('Ctrl Pts',(3.,-6.08767497843372,33.5306623697168));
#50215=CARTESIAN_POINT('Ctrl Pts',(2.93740375632004,-6.08767497843372,33.5306623697168));
#50216=CARTESIAN_POINT('Ctrl Pts',(2.87565789134417,-6.09830402968066,33.5286044607783));
#50217=CARTESIAN_POINT('Ctrl Pts',(2.7340154507069,-6.14671873130704,33.5182630464583));
#50218=CARTESIAN_POINT('Ctrl Pts',(2.65923300361173,-6.19233182892453,33.5081456447411));
#50219=CARTESIAN_POINT('Ctrl Pts',(2.52172868443329,-6.31191640618344,33.474380862772));
#50220=CARTESIAN_POINT('Ctrl Pts',(2.46172409835087,-6.38885879373992,33.4491371944454));
#50221=CARTESIAN_POINT('Ctrl Pts',(2.39060701245703,-6.51897766283339,33.3880551373259));
#50222=CARTESIAN_POINT('Ctrl Pts',(2.36956327353233,-6.57078939327562,33.3592077605039));
#50223=CARTESIAN_POINT('Ctrl Pts',(2.34883638351776,-6.64971896474131,33.3034617254313));
#50224=CARTESIAN_POINT('Ctrl Pts',(2.3439753226196,-6.67778206838815,33.2810310563229));
#50225=CARTESIAN_POINT('Ctrl Pts',(2.34028669329881,-6.72781049660138,33.2352666165328));
#50226=CARTESIAN_POINT('Ctrl Pts',(2.34077606978153,-6.74979295500869,33.2127109504232));
#50227=CARTESIAN_POINT('Ctrl Pts',(2.34680248319783,-6.79615911042747,33.1594014885423));
#50228=CARTESIAN_POINT('Ctrl Pts',(2.35349632945343,-6.81939902656572,33.1284582077866));
#50229=CARTESIAN_POINT('Ctrl Pts',(2.38103390803268,-6.87804712505278,33.0394879640942));
#50230=CARTESIAN_POINT('Ctrl Pts',(2.40863932166365,-6.90772580028372,32.9805175921408));
#50231=CARTESIAN_POINT('Ctrl Pts',(2.49309498094623,-6.96395620747035,32.8471138586884));
#50232=CARTESIAN_POINT('Ctrl Pts',(2.55769731566228,-6.98583852522132,32.7741439823312));
#50233=CARTESIAN_POINT('Ctrl Pts',(2.69643706868993,-7.01339895805738,32.6694564844565));
#50234=CARTESIAN_POINT('Ctrl Pts',(2.76629587634983,-7.0213517213066,32.6325650487793));
#50235=CARTESIAN_POINT('Ctrl Pts',(2.89345183041014,-7.02914761950449,32.5954348113669));
#50236=CARTESIAN_POINT('Ctrl Pts',(2.94650789475066,-7.03066236971681,32.5876749784337));
#50237=CARTESIAN_POINT('Ctrl Pts',(3.,-7.03066236971681,32.5876749784337));
#50238=CARTESIAN_POINT('',(3.,-3.62392225358105,31.2199377644202));
#50239=CARTESIAN_POINT('Origin',(3.,4.17193000900063,30.6719300090006));
#50240=CARTESIAN_POINT('',(3.65899840720327,6.73112601132474,33.2311260113247));
#50241=CARTESIAN_POINT('',(3.,7.0306623697168,32.5876749784337));
#50242=CARTESIAN_POINT('Ctrl Pts',(3.65899840720327,6.73112601132474,33.2311260113247));
#50243=CARTESIAN_POINT('Ctrl Pts',(3.65899840720327,6.7354593368928,33.2267926857567));
#50244=CARTESIAN_POINT('Ctrl Pts',(3.65891512098013,6.73974331606797,33.2224121818583));
#50245=CARTESIAN_POINT('Ctrl Pts',(3.65781547543883,6.76770757636843,33.1931745733099));
#50246=CARTESIAN_POINT('Ctrl Pts',(3.65428413830506,6.7896669413199,33.1671050240486));
#50247=CARTESIAN_POINT('Ctrl Pts',(3.63870034113715,6.84187441417481,33.0972791835609));
#50248=CARTESIAN_POINT('Ctrl Pts',(3.62306713231026,6.86897171042236,33.0527898875676));
#50249=CARTESIAN_POINT('Ctrl Pts',(3.56551968033943,6.93231573116172,32.9308889246305));
#50250=CARTESIAN_POINT('Ctrl Pts',(3.51273077708478,6.96030777397002,32.8539988734892));
#50251=CARTESIAN_POINT('Ctrl Pts',(3.38847748053925,6.99899785132441,32.7283829770697));
#50252=CARTESIAN_POINT('Ctrl Pts',(3.31889126238351,7.01124568545061,32.6772205194953));
#50253=CARTESIAN_POINT('Ctrl Pts',(3.1753255784899,7.02602030562166,32.6113437863197));
#50254=CARTESIAN_POINT('Ctrl Pts',(3.10504775292266,7.02961884290778,32.5928825083459));
#50255=CARTESIAN_POINT('Ctrl Pts',(3.0216026766366,7.03059936386323,32.587990297225));
#50256=CARTESIAN_POINT('Ctrl Pts',(3.01078870740021,7.0306623697168,32.5876749784337));
#50257=CARTESIAN_POINT('Ctrl Pts',(3.,7.0306623697168,32.5876749784337));
#50258=CARTESIAN_POINT('',(3.,6.08767497843373,33.5306623697168));
#50259=CARTESIAN_POINT('Ctrl Pts',(3.,6.08767497843373,33.5306623697168));
#50260=CARTESIAN_POINT('Ctrl Pts',(3.01771871221484,6.08767497843373,33.5306623697168));
#50261=CARTESIAN_POINT('Ctrl Pts',(3.03548526784969,6.08852552424608,33.5304927152597));
#50262=CARTESIAN_POINT('Ctrl Pts',(3.12997701049221,6.09763707361585,33.5286602673591));
#50263=CARTESIAN_POINT('Ctrl Pts',(3.20348422043877,6.12080466665807,33.5241018511828));
#50264=CARTESIAN_POINT('Ctrl Pts',(3.34957484663778,6.19739536479966,33.5063721276838));
#50265=CARTESIAN_POINT('Ctrl Pts',(3.41865686125508,6.2540323110953,33.4921652747427));
#50266=CARTESIAN_POINT('Ctrl Pts',(3.53708659094318,6.38703324760799,33.4483236156805));
#50267=CARTESIAN_POINT('Ctrl Pts',(3.58549288386577,6.46524437901786,33.4174179808017));
#50268=CARTESIAN_POINT('Ctrl Pts',(3.63325765640775,6.58179850667398,33.3511743356787));
#50269=CARTESIAN_POINT('Ctrl Pts',(3.6449718023722,6.62056029041712,33.325635980606));
#50270=CARTESIAN_POINT('Ctrl Pts',(3.65660045499355,6.68331519828023,33.2761367819232));
#50271=CARTESIAN_POINT('Ctrl Pts',(3.65899840720327,6.7078407754763,33.2544112471732));
#50272=CARTESIAN_POINT('Ctrl Pts',(3.65899840720327,6.73112601132474,33.2311260113247));
#50273=CARTESIAN_POINT('Ctrl Pts',(3.,7.0306623697168,32.5876749784337));
#50274=CARTESIAN_POINT('Ctrl Pts',(2.93740375631998,7.0306623697168,32.5876749784337));
#50275=CARTESIAN_POINT('Ctrl Pts',(2.87565789134411,7.02860446077826,32.5983040296807));
#50276=CARTESIAN_POINT('Ctrl Pts',(2.73401545070677,7.01826304645831,32.6467187313071));
#50277=CARTESIAN_POINT('Ctrl Pts',(2.65923300361162,7.0081456447411,32.6923318289246));
#50278=CARTESIAN_POINT('Ctrl Pts',(2.52172868443319,6.97438086277194,32.8119164061835));
#50279=CARTESIAN_POINT('Ctrl Pts',(2.46172409835081,6.94913719444534,32.88885879374));
#50280=CARTESIAN_POINT('Ctrl Pts',(2.39060701245699,6.88805513732588,33.0189776628335));
#50281=CARTESIAN_POINT('Ctrl Pts',(2.36956327353232,6.85920776050379,33.0707893932757));
#50282=CARTESIAN_POINT('Ctrl Pts',(2.34883638351776,6.80346172543131,33.1497189647413));
#50283=CARTESIAN_POINT('Ctrl Pts',(2.34397532261961,6.78103105632281,33.1777820683882));
#50284=CARTESIAN_POINT('Ctrl Pts',(2.34028669329882,6.73526661653279,33.2278104966014));
#50285=CARTESIAN_POINT('Ctrl Pts',(2.34077606978155,6.71271095042312,33.2497929550087));
#50286=CARTESIAN_POINT('Ctrl Pts',(2.34680248319785,6.65940148854226,33.2961591104275));
#50287=CARTESIAN_POINT('Ctrl Pts',(2.35349632945345,6.62845820778652,33.3193990265657));
#50288=CARTESIAN_POINT('Ctrl Pts',(2.38103390803271,6.53948796409412,33.3780471250528));
#50289=CARTESIAN_POINT('Ctrl Pts',(2.40863932166368,6.48051759214078,33.4077258002837));
#50290=CARTESIAN_POINT('Ctrl Pts',(2.49309498094631,6.34711385868828,33.4639562074704));
#50291=CARTESIAN_POINT('Ctrl Pts',(2.55769731566239,6.27414398233109,33.4858385252213));
#50292=CARTESIAN_POINT('Ctrl Pts',(2.69643706869003,6.16945648445639,33.5133989580574));
#50293=CARTESIAN_POINT('Ctrl Pts',(2.76629587634994,6.13256504877923,33.5213517213066));
#50294=CARTESIAN_POINT('Ctrl Pts',(2.89345183041017,6.09543481136693,33.5291476195045));
#50295=CARTESIAN_POINT('Ctrl Pts',(2.94650789475069,6.08767497843373,33.5306623697168));
#50296=CARTESIAN_POINT('Ctrl Pts',(3.,6.08767497843373,33.5306623697168));
#50297=CARTESIAN_POINT('',(3.,4.7199377644202,30.1239222535811));
#50298=CARTESIAN_POINT('Origin',(3.,0.,26.5));
#50299=CARTESIAN_POINT('',(3.,-1.13892152320704E-15,35.8));
#50300=CARTESIAN_POINT('Origin',(3.,-1.27363267111325E-15,36.9));
#50301=CARTESIAN_POINT('Origin',(3.,0.,26.5));
#50302=CARTESIAN_POINT('Origin',(3.,0.,26.5));
#50303=CARTESIAN_POINT('Origin',(3.,0.,26.5));
#50304=CARTESIAN_POINT('Origin',(3.,0.,26.5));
#50305=CARTESIAN_POINT('Origin',(3.,0.,26.5));
#50306=CARTESIAN_POINT('Origin',(1.05,0.,26.5));
#50307=CARTESIAN_POINT('',(1.3,-0.46,26.5));
#50308=CARTESIAN_POINT('Origin',(1.3,0.,26.5));
#50309=CARTESIAN_POINT('',(1.05,-0.46,26.5));
#50310=CARTESIAN_POINT('Origin',(1.3,0.46,26.5));
#76625=UNCERTAINTY_MEASURE_WITH_UNIT(LENGTH_MEASURE(0.001),#76661,
'DISTANCE_ACCURACY_VALUE',
'Maximum model space distance between geometric entities at asserted c
onnectivities');
#76638=UNCERTAINTY_MEASURE_WITH_UNIT(LENGTH_MEASURE(0.001),#76661,
'DISTANCE_ACCURACY_VALUE',
'Maximum model space distance between geometric entities at asserted c
onnectivities');
#76647=(
GEOMETRIC_REPRESENTATION_CONTEXT(3)
GLOBAL_UNCERTAINTY_ASSIGNED_CONTEXT((#76625))
GLOBAL_UNIT_ASSIGNED_CONTEXT((#76661,#76663,#76664))
REPRESENTATION_CONTEXT('','3D')
);
#76660=(
GEOMETRIC_REPRESENTATION_CONTEXT(3)
GLOBAL_UNCERTAINTY_ASSIGNED_CONTEXT((#76638))
GLOBAL_UNIT_ASSIGNED_CONTEXT((#76661,#76663,#76664))
REPRESENTATION_CONTEXT('','3D')
);
#76661=(
LENGTH_UNIT()
NAMED_UNIT(*)
SI_UNIT(.CENTI.,.METRE.)
);
#76663=(
NAMED_UNIT(*)
PLANE_ANGLE_UNIT()
SI_UNIT($,.RADIAN.)
);
#76664=(
NAMED_UNIT(*)
SI_UNIT($,.STERADIAN.)
SOLID_ANGLE_UNIT()
);
#76673=SHAPE_DEFINITION_REPRESENTATION(#76694,#76743);
#76694=PRODUCT_DEFINITION_SHAPE('',$,#76765);
#76743=SHAPE_REPRESENTATION('',(#27825),#76647);
#76756=PRODUCT_DEFINITION_CONTEXT('part definition',#76821,'design');
#76765=PRODUCT_DEFINITION('2026-10-26-11-12-58-000',
'09_Quill_Handwheel_D230_4_Spoke',#76786,#76756);
#76786=PRODUCT_DEFINITION_FORMATION('',$,#76831);
#76821=APPLICATION_CONTEXT(
'Core Data for Automotive Mechanical Design Process');
#76822=PRODUCT_CONTEXT('part definition',#76821,'mechanical');
#76831=PRODUCT('2026-10-26-11-12-58-000',
'09_Quill_Handwheel_D230_4_Spoke',$,(#76822));
#76893=COLOUR_RGB('Sky Blue',0.24,0.69,0.87);
#76894=FILL_AREA_STYLE_COLOUR('',#76893);
#76895=FILL_AREA_STYLE('',(#76894));
#76896=SURFACE_STYLE_FILL_AREA(#76895);
#76897=SURFACE_SIDE_STYLE('',(#76896));
#76898=SURFACE_STYLE_USAGE(.BOTH.,#76897);
#76899=PRESENTATION_STYLE_ASSIGNMENT((#76898));
ENDSEC;
END-ISO-10303-21;
